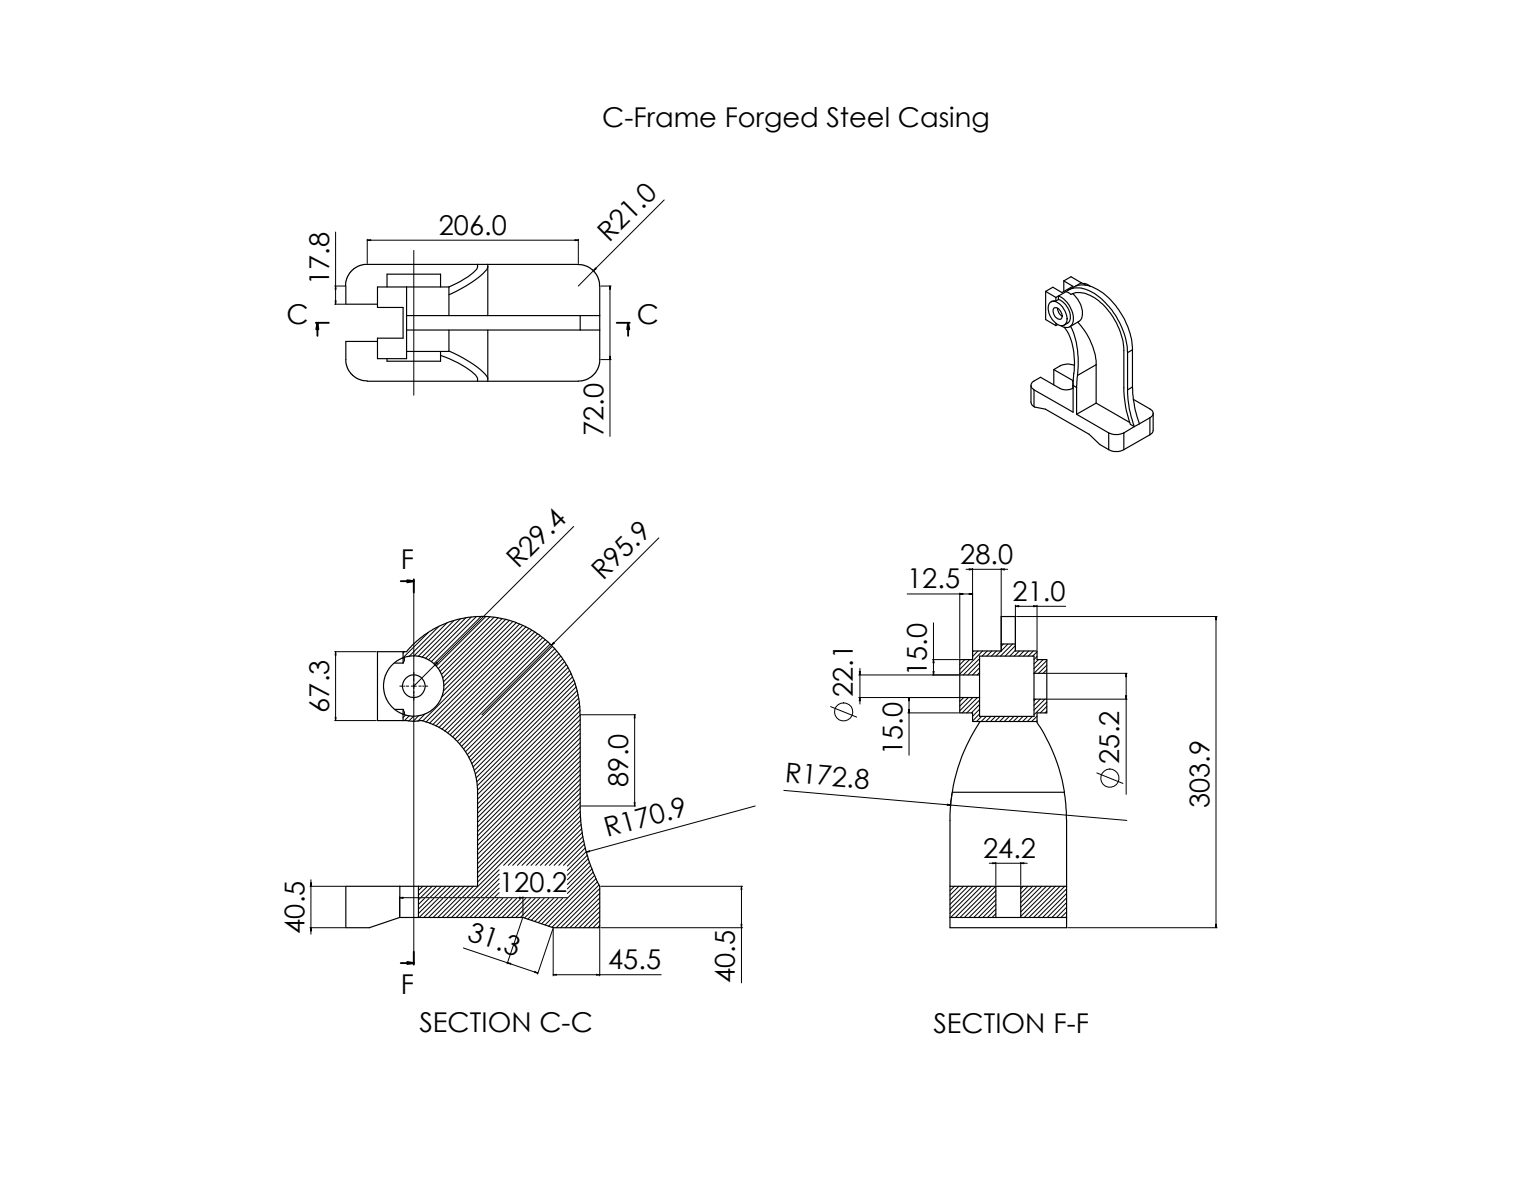
ISO-10303-21;
HEADER;
FILE_DESCRIPTION (('STEP AP214'),
    '1' );
FILE_NAME ('C-Frame Forged Steel Casing.step',
    '2026-10-21T18:33:49',
    ( '' ),
    ( '' ),
    'SwSTEP 2.0',
    'SolidWorks 2025',
    '' );
FILE_SCHEMA (( 'AUTOMOTIVE_DESIGN' ));
ENDSEC;

DATA;
#4=VERTEX_POINT ( 'NONE', #5573 ) ;
#12=DIRECTION ( 'NONE',  ( -0.000000000000000000, -0.000000000000000000, -1.000000000000000000 ) ) ;
#27=ADVANCED_FACE ( 'NONE', ( #4362 ), #9999, .F. ) ;
#28=VECTOR ( 'NONE', #11841, 1000.000000000000000 ) ;
#45=AXIS2_PLACEMENT_3D ( 'NONE', #14996, #2189, #7901 ) ;
#46=ORIENTED_EDGE ( 'NONE', *, *, #11434, .F. ) ;
#52=DIRECTION ( 'NONE',  ( -1.000000000000000000, -0.000000000000000000, -0.000000000000000000 ) ) ;
#63=CARTESIAN_POINT ( 'NONE',  ( -9.730036491473859073, 24.55694320255973651, 41.56001028271458608 ) ) ;
#65=ORIENTED_EDGE ( 'NONE', *, *, #13144, .F. ) ;
#81=ADVANCED_FACE ( 'NONE', ( #3143 ), #14460, .T. ) ;
#90=DIRECTION ( 'NONE',  ( -0.000000000000000000, 0.000000000000000000, -1.000000000000000000 ) ) ;
#91=LINE ( 'NONE', #5786, #7353 ) ;
#111=AXIS2_PLACEMENT_3D ( 'NONE', #807, #12215, #17823 ) ;
#116=EDGE_CURVE ( 'NONE', #6374, #8001, #17153, .T. ) ;
#139=CARTESIAN_POINT ( 'NONE',  ( -127.5926225674731711, 57.88796029049329661, -26.35917033480641436 ) ) ;
#144=ADVANCED_FACE ( 'NONE', ( #11916 ), #17609, .T. ) ;
#164=DIRECTION ( 'NONE',  ( -1.000000000000000000, 0.000000000000000000, 0.000000000000000000 ) ) ;
#170=FACE_OUTER_BOUND ( 'NONE', #6777, .T. ) ;
#173=VECTOR ( 'NONE', #14749, 1000.000000000000000 ) ;
#176=DIRECTION ( 'NONE',  ( 0.000000000000000000, 1.000000000000000000, 0.000000000000000000 ) ) ;
#177=ORIENTED_EDGE ( 'NONE', *, *, #14769, .T. ) ;
#183=CARTESIAN_POINT ( 'NONE',  ( -70.85175816390371040, -141.5628872026273086, -18.23991632971910803 ) ) ;
#186=CARTESIAN_POINT ( 'NONE',  ( 49.38736944425944841, -141.5628872026273086, -57.00000000000000000 ) ) ;
#188=DIRECTION ( 'NONE',  ( 0.000000000000000000, 0.000000000000000000, 1.000000000000000000 ) ) ;
#203=FACE_OUTER_BOUND ( 'NONE', #17910, .T. ) ;
#204=FACE_OUTER_BOUND ( 'NONE', #12195, .T. ) ;
#205=CARTESIAN_POINT ( 'NONE',  ( -64.09025127992788384, 50.58224449241410525, 35.00000000000000000 ) ) ;
#225=ORIENTED_EDGE ( 'NONE', *, *, #7011, .F. ) ;
#229=EDGE_CURVE ( 'NONE', #6748, #3936, #16550, .T. ) ;
#231=ORIENTED_EDGE ( 'NONE', *, *, #17262, .F. ) ;
#234=DIRECTION ( 'NONE',  ( 0.000000000000000000, 0.000000000000000000, 1.000000000000000000 ) ) ;
#236=ORIENTED_EDGE ( 'NONE', *, *, #5271, .F. ) ;
#241=ORIENTED_EDGE ( 'NONE', *, *, #15088, .F. ) ;
#244=EDGE_CURVE ( 'NONE', #4575, #11504, #16586, .T. ) ;
#255=EDGE_CURVE ( 'NONE', #17238, #6285, #13006, .T. ) ;
#263=ORIENTED_EDGE ( 'NONE', *, *, #18181, .T. ) ;
#266=CARTESIAN_POINT ( 'NONE',  ( -37.39678785461407529, 56.02900023377289074, 23.03959524935876857 ) ) ;
#268=DIRECTION ( 'NONE',  ( -0.000000000000000000, -0.000000000000000000, -1.000000000000000000 ) ) ;
#270=ORIENTED_EDGE ( 'NONE', *, *, #16707, .F. ) ;
#271=CARTESIAN_POINT ( 'NONE',  ( -66.92930002414082935, 60.44851893123529152, 25.00000000000000000 ) ) ;
#284=DIRECTION ( 'NONE',  ( 0.000000000000000000, 0.000000000000000000, 1.000000000000000000 ) ) ;
#293=VERTEX_POINT ( 'NONE', #8174 ) ;
#299=VERTEX_POINT ( 'NONE', #17149 ) ;
#301=DIRECTION ( 'NONE',  ( 0.000000000000000000, 0.000000000000000000, -1.000000000000000000 ) ) ;
#302=CARTESIAN_POINT ( 'NONE',  ( 105.4583593777967963, -32.62665103886256190, -7.000000000000010658 ) ) ;
#306=ORIENTED_EDGE ( 'NONE', *, *, #1227, .F. ) ;
#318=AXIS2_PLACEMENT_3D ( 'NONE', #739, #6431, #16426 ) ;
#325=CARTESIAN_POINT ( 'NONE',  ( -69.66239992860627694, 84.22855780814606419, 37.50000000000000000 ) ) ;
#330=ORIENTED_EDGE ( 'NONE', *, *, #16668, .T. ) ;
#331=EDGE_CURVE ( 'NONE', #1479, #11856, #14263, .T. ) ;
#337=AXIS2_PLACEMENT_3D ( 'NONE', #17527, #14630, #13242 ) ;
#355=FACE_OUTER_BOUND ( 'NONE', #8735, .T. ) ;
#357=CARTESIAN_POINT ( 'NONE',  ( -57.08002265617300708, 84.22855780814606419, 37.50000000000000000 ) ) ;
#367=CARTESIAN_POINT ( 'NONE',  ( -66.14751942900640813, 58.73266222548429027, 25.00000000000001066 ) ) ;
#375=CYLINDRICAL_SURFACE ( 'NONE', #9052, 85.91469608272775815 ) ;
#378=CARTESIAN_POINT ( 'NONE',  ( -71.20965894365861004, 109.9770744052236324, 22.40029077787859890 ) ) ;
#384=DIRECTION ( 'NONE',  ( -0.000000000000000000, 1.000000000000000000, -1.200240087506842815E-16 ) ) ;
#390=DIRECTION ( 'NONE',  ( 0.000000000000000000, 0.000000000000000000, 1.000000000000000000 ) ) ;
#394=CIRCLE ( 'NONE', #2180, 3.999999999999982681 ) ;
#395=AXIS2_PLACEMENT_3D ( 'NONE', #4110, #9813, #15514 ) ;
#397=CARTESIAN_POINT ( 'NONE',  ( -50.06979403241810900, 50.58224449241409104, -26.91246033477409583 ) ) ;
#399=ORIENTED_EDGE ( 'NONE', *, *, #757, .T. ) ;
#412=AXIS2_PLACEMENT_3D ( 'NONE', #18211, #5379, #6987 ) ;
#414=EDGE_CURVE ( 'NONE', #2953, #996, #7597, .T. ) ;
#416=EDGE_CURVE ( 'NONE', #17198, #9318, #10399, .T. ) ;
#420=VECTOR ( 'NONE', #9508, 1000.000000000000000 ) ;
#426=DIRECTION ( 'NONE',  ( -0.000000000000000000, -0.000000000000000000, -1.000000000000000000 ) ) ;
#429=ORIENTED_EDGE ( 'NONE', *, *, #6145, .F. ) ;
#430=VECTOR ( 'NONE', #5454, 1000.000000000000000 ) ;
#433=CARTESIAN_POINT ( 'NONE',  ( 15.23320273812466574, -111.0842361345572158, 57.00000000000000000 ) ) ;
#443=( LENGTH_UNIT ( ) NAMED_UNIT ( * ) SI_UNIT ( .MILLI., .METRE. ) );
#452=AXIS2_PLACEMENT_3D ( 'NONE', #2320, #3822, #12451 ) ;
#457=EDGE_CURVE ( 'NONE', #3111, #2581, #12721, .T. ) ;
#468=EDGE_CURVE ( 'NONE', #18251, #15291, #12961, .T. ) ;
#476=DIRECTION ( 'NONE',  ( 0.000000000000000000, 0.000000000000000000, -1.000000000000000000 ) ) ;
#481=CARTESIAN_POINT ( 'NONE',  ( 113.3630170098442989, -111.0842361345572158, -3.000000000000000000 ) ) ;
#482=ORIENTED_EDGE ( 'NONE', *, *, #4046, .F. ) ;
#485=EDGE_CURVE ( 'NONE', #2052, #18444, #13583, .T. ) ;
#486=ORIENTED_EDGE ( 'NONE', *, *, #1405, .F. ) ;
#487=ADVANCED_FACE ( 'NONE', ( #16560 ), #14878, .T. ) ;
#491=CARTESIAN_POINT ( 'NONE',  ( -38.40665361001209988, 55.34834135440265612, -23.54080219878014546 ) ) ;
#492=CARTESIAN_POINT ( 'NONE',  ( -102.4618227840623774, -151.5628872026273086, 57.00000000000000000 ) ) ;
#496=CARTESIAN_POINT ( 'NONE',  ( 276.3098885457529832, -32.62665103886256190, 7.000000000000010658 ) ) ;
#503=ORIENTED_EDGE ( 'NONE', *, *, #14484, .F. ) ;
#504=ORIENTED_EDGE ( 'NONE', *, *, #2706, .T. ) ;
#505=VERTEX_POINT ( 'NONE', #2158 ) ;
#510=DIRECTION ( 'NONE',  ( -0.000000000000000000, 0.000000000000000000, 1.000000000000000000 ) ) ;
#523=EDGE_LOOP ( 'NONE', ( #7059, #9577, #8331, #14594 ) ) ;
#530=CARTESIAN_POINT ( 'NONE',  ( -66.63376473465912397, -19.34983604512935429, 57.00000000000000000 ) ) ;
#532=CARTESIAN_POINT ( 'NONE',  ( -67.59262256747319952, 110.5691553257988460, -30.35917033480640370 ) ) ;
#535=VERTEX_POINT ( 'NONE', #769 ) ;
#537=DIRECTION ( 'NONE',  ( 0.000000000000000000, 1.000000000000000000, 0.000000000000000000 ) ) ;
#543=ORIENTED_EDGE ( 'NONE', *, *, #11265, .T. ) ;
#546=DIRECTION ( 'NONE',  ( 1.000000000000000000, 0.000000000000000000, 0.000000000000000000 ) ) ;
#550=CARTESIAN_POINT ( 'NONE',  ( 124.5381772159375942, -151.5628872026272802, 57.00000000000000000 ) ) ;
#552=CARTESIAN_POINT ( 'NONE',  ( -86.44887054343442401, 84.22855780814606419, -15.00000000000000711 ) ) ;
#556=CARTESIAN_POINT ( 'NONE',  ( -76.09645744896180020, 61.84763831329342310, -26.96898856272271772 ) ) ;
#559=ORIENTED_EDGE ( 'NONE', *, *, #11791, .T. ) ;
#561=ADVANCED_FACE ( 'NONE', ( #13672, #6655 ), #7775, .T. ) ;
#565=VERTEX_POINT ( 'NONE', #10486 ) ;
#570=ADVANCED_FACE ( 'NONE', ( #7868 ), #12377, .F. ) ;
#573=VERTEX_POINT ( 'NONE', #14965 ) ;
#588=CARTESIAN_POINT ( 'NONE',  ( -127.5926225674731711, 57.88796029049329661, -22.35917033480642502 ) ) ;
#591=ORIENTED_EDGE ( 'NONE', *, *, #12155, .F. ) ;
#608=CARTESIAN_POINT ( 'NONE',  ( -66.46434123065944277, 108.9297695310272331, 25.00000000000000000 ) ) ;
#609=ORIENTED_EDGE ( 'NONE', *, *, #8356, .T. ) ;
#611=CARTESIAN_POINT ( 'NONE',  ( -67.59262256747319952, 110.5691553257988460, 26.35917033480641436 ) ) ;
#615=AXIS2_PLACEMENT_3D ( 'NONE', #18506, #12902, #11404 ) ;
#632=CARTESIAN_POINT ( 'NONE',  ( 15.23320273812466041, -46.83756720124470263, -57.00000000000000000 ) ) ;
#637=DIRECTION ( 'NONE',  ( -1.000000000000000000, -0.000000000000000000, -0.000000000000000000 ) ) ;
#656=CARTESIAN_POINT ( 'NONE',  ( -75.85991620623855169, 61.64845565236244340, -24.98030658468874066 ) ) ;
#661=AXIS2_PLACEMENT_3D ( 'NONE', #357, #3872, #9580 ) ;
#670=DIRECTION ( 'NONE',  ( -0.000000000000000000, 1.000000000000000000, -0.000000000000000000 ) ) ;
#678=EDGE_CURVE ( 'NONE', #17304, #14302, #10606, .T. ) ;
#679=CYLINDRICAL_SURFACE ( 'NONE', #15266, 180.8515291679561585 ) ;
#680=DIRECTION ( 'NONE',  ( 1.000000000000000000, 2.062304371594500494E-16, -0.000000000000000000 ) ) ;
#685=ORIENTED_EDGE ( 'NONE', *, *, #12458, .T. ) ;
#687=EDGE_CURVE ( 'NONE', #18482, #6976, #11196, .T. ) ;
#707=ORIENTED_EDGE ( 'NONE', *, *, #4942, .F. ) ;
#712=ADVANCED_FACE ( 'NONE', ( #1423 ), #18070, .F. ) ;
#713=CARTESIAN_POINT ( 'NONE',  ( 49.38736944425944841, -141.5628872026273086, -57.00000000000000000 ) ) ;
#721=ORIENTED_EDGE ( 'NONE', *, *, #229, .F. ) ;
#726=CARTESIAN_POINT ( 'NONE',  ( 5.233202738124663966, -15.18076580469977621, 54.12731639097741976 ) ) ;
#727=EDGE_CURVE ( 'NONE', #299, #9555, #15255, .T. ) ;
#739=CARTESIAN_POINT ( 'NONE',  ( -127.5926225674731711, 57.88796029049329661, 26.35917033480641436 ) ) ;
#741=PLANE ( 'NONE',  #2390 ) ;
#748=VERTEX_POINT ( 'NONE', #8151 ) ;
#752=CARTESIAN_POINT ( 'NONE',  ( -66.09157170483439359, 57.23989889526016839, 25.00000000000000711 ) ) ;
#757=EDGE_CURVE ( 'NONE', #8476, #13829, #13867, .T. ) ;
#758=CARTESIAN_POINT ( 'NONE',  ( -73.90024509548729270, 60.14960425286541579, -23.04802554496307820 ) ) ;
#769=CARTESIAN_POINT ( 'NONE',  ( -92.59262256747321373, 117.8748711238780373, -35.00000000000000000 ) ) ;
#777=LINE ( 'NONE', #16857, #3625 ) ;
#788=DIRECTION ( 'NONE',  ( 0.000000000000000000, 0.000000000000000000, 1.000000000000000000 ) ) ;
#791=CARTESIAN_POINT ( 'NONE',  ( -92.59262256747319952, 57.88796029049329661, -26.35917033480641436 ) ) ;
#798=DIRECTION ( 'NONE',  ( -0.000000000000000000, -0.000000000000000000, -1.000000000000000000 ) ) ;
#802=ADVANCED_FACE ( 'NONE', ( #10295 ), #10201, .F. ) ;
#804=CARTESIAN_POINT ( 'NONE',  ( -102.4618227840623774, -151.5628872026273086, -36.00000000000000000 ) ) ;
#806=ORIENTED_EDGE ( 'NONE', *, *, #924, .F. ) ;
#807=CARTESIAN_POINT ( 'NONE',  ( -57.08002265617300708, 84.22855780814606419, -35.00000000000000711 ) ) ;
#838=CARTESIAN_POINT ( 'NONE',  ( -64.09025127992788384, 50.58224449241410525, 35.00000000000000000 ) ) ;
#843=CARTESIAN_POINT ( 'NONE',  ( -123.4618227840623632, -151.5628872026273086, -18.23991632971910093 ) ) ;
#847=FACE_OUTER_BOUND ( 'NONE', #13419, .T. ) ;
#862=ORIENTED_EDGE ( 'NONE', *, *, #18382, .T. ) ;
#870=AXIS2_PLACEMENT_3D ( 'NONE', #11609, #12763, #7219 ) ;
#880=CARTESIAN_POINT ( 'NONE',  ( -123.4618227840623632, -111.0842361345572158, 57.00000000000000000 ) ) ;
#882=AXIS2_PLACEMENT_3D ( 'NONE', #13146, #12986, #164 ) ;
#883=CARTESIAN_POINT ( 'NONE',  ( -72.81448312412459245, 109.0309132574646469, -22.65846447477133196 ) ) ;
#885=VERTEX_POINT ( 'NONE', #5803 ) ;
#890=EDGE_CURVE ( 'NONE', #6749, #1925, #15737, .T. ) ;
#892=AXIS2_PLACEMENT_3D ( 'NONE', #1155, #10880, #1247 ) ;
#898=VECTOR ( 'NONE', #16815, 1000.000000000000000 ) ;
#902=B_SPLINE_CURVE_WITH_KNOTS ( 'NONE', 3,
 ( #11513, #2811, #7287, #2981 ),
 .UNSPECIFIED., .F., .F.,
 ( 4, 4 ),
 ( 0.000000000000000000, 0.002699315152504066541 ),
 .UNSPECIFIED. ) ;
#906=CARTESIAN_POINT ( 'NONE',  ( -67.59262256747319952, 110.5691553257988460, 30.35917033480640370 ) ) ;
#908=CARTESIAN_POINT ( 'NONE',  ( 9.543663295069050534, 56.41207303426870112, 7.000000000000010658 ) ) ;
#916=DIRECTION ( 'NONE',  ( -1.000000000000000000, 0.000000000000000000, -0.000000000000000000 ) ) ;
#924=EDGE_CURVE ( 'NONE', #6138, #3111, #9170, .T. ) ;
#927=CARTESIAN_POINT ( 'NONE',  ( -66.75350761719796822, 56.49772428296282811, 24.14382665953563745 ) ) ;
#929=CARTESIAN_POINT ( 'NONE',  ( -66.56081925660646448, 59.51305259755623212, -27.99999999999999645 ) ) ;
#931=EDGE_CURVE ( 'NONE', #505, #8038, #6442, .T. ) ;
#934=EDGE_CURVE ( 'NONE', #15744, #1208, #5522, .T. ) ;
#938=ORIENTED_EDGE ( 'NONE', *, *, #890, .F. ) ;
#946=DIRECTION ( 'NONE',  ( -0.000000000000000000, 0.000000000000000000, 1.000000000000000000 ) ) ;
#951=ADVANCED_FACE ( 'NONE', ( #5030 ), #13463, .F. ) ;
#963=CARTESIAN_POINT ( 'NONE',  ( -123.4618227840623632, -151.5628872026273086, 57.00000000000000000 ) ) ;
#982=VECTOR ( 'NONE', #13264, 1000.000000000000000 ) ;
#986=ORIENTED_EDGE ( 'NONE', *, *, #12489, .F. ) ;
#987=CARTESIAN_POINT ( 'NONE',  ( -74.24593559006332555, 108.0616442416786640, -23.22608149512904063 ) ) ;
#994=DIRECTION ( 'NONE',  ( -0.000000000000000000, -1.000000000000000000, -0.000000000000000000 ) ) ;
#996=VERTEX_POINT ( 'NONE', #13656 ) ;
#1007=CARTESIAN_POINT ( 'NONE',  ( -123.4618227840623632, -111.0842361345572158, 57.00000000000000000 ) ) ;
#1008=ORIENTED_EDGE ( 'NONE', *, *, #10694, .T. ) ;
#1010=CARTESIAN_POINT ( 'NONE',  ( -112.5926225674731995, 50.58224449241410525, 35.00000000000000000 ) ) ;
#1018=AXIS2_PLACEMENT_3D ( 'NONE', #18076, #8156, #2447 ) ;
#1021=FACE_OUTER_BOUND ( 'NONE', #2125, .T. ) ;
#1023=VECTOR ( 'NONE', #12613, 1000.000000000000000 ) ;
#1026=CARTESIAN_POINT ( 'NONE',  ( 103.5381772159376084, -151.5628872026272802, 57.00000000000000000 ) ) ;
#1027=AXIS2_PLACEMENT_3D ( 'NONE', #13141, #17251, #1911 ) ;
#1029=CARTESIAN_POINT ( 'NONE',  ( -67.37336793441032512, 56.72162401922281560, 22.91103267187422787 ) ) ;
#1038=CARTESIAN_POINT ( 'NONE',  ( -0.000000000000000000, -111.0842361345572158, -3.000000000000000000 ) ) ;
#1040=ORIENTED_EDGE ( 'NONE', *, *, #11176, .F. ) ;
#1041=EDGE_CURVE ( 'NONE', #13411, #11585, #10588, .T. ) ;
#1049=ORIENTED_EDGE ( 'NONE', *, *, #15194, .T. ) ;
#1054=AXIS2_PLACEMENT_3D ( 'NONE', #5183, #18105, #10990 ) ;
#1059=CARTESIAN_POINT ( 'NONE',  ( -64.09025127992789805, 117.8748711238780089, 7.000000000000010658 ) ) ;
#1063=EDGE_CURVE ( 'NONE', #3060, #4, #4507, .T. ) ;
#1067=VECTOR ( 'NONE', #16551, 1000.000000000000000 ) ;
#1069=CARTESIAN_POINT ( 'NONE',  ( -112.5926225674731853, 50.58224449241410525, 15.00000000000004796 ) ) ;
#1072=DIRECTION ( 'NONE',  ( 0.000000000000000000, 0.000000000000000000, 1.000000000000000000 ) ) ;
#1080=EDGE_LOOP ( 'NONE', ( #7717, #7540 ) ) ;
#1083=VECTOR ( 'NONE', #15801, 1000.000000000000000 ) ;
#1084=VECTOR ( 'NONE', #5911, 1000.000000000000000 ) ;
#1086=CARTESIAN_POINT ( 'NONE',  ( 9.543663295069050534, 56.41207303426870112, -7.000000000000010658 ) ) ;
#1091=ORIENTED_EDGE ( 'NONE', *, *, #16945, .T. ) ;
#1092=CARTESIAN_POINT ( 'NONE',  ( -100.4870060002411805, -151.5628872026273086, 18.23991632971911514 ) ) ;
#1096=CARTESIAN_POINT ( 'NONE',  ( -75.82627924895463423, 106.8366279053472283, -27.81200583293166417 ) ) ;
#1104=ORIENTED_EDGE ( 'NONE', *, *, #9720, .F. ) ;
#1105=DIRECTION ( 'NONE',  ( -0.9475106458593564041, 0.3197242186372270534, -0.000000000000000000 ) ) ;
#1113=CARTESIAN_POINT ( 'NONE',  ( 5.233202738124664855, -19.34983604512936495, -54.79921157549230770 ) ) ;
#1114=CARTESIAN_POINT ( 'NONE',  ( -6.009442422294567265, 35.67642109510119752, 36.02332778080708664 ) ) ;
#1123=PLANE ( 'NONE',  #1879 ) ;
#1124=LINE ( 'NONE', #7948, #12683 ) ;
#1127=CARTESIAN_POINT ( 'NONE',  ( -45.07766827056850190, 51.92519128693054142, 25.99195503995988688 ) ) ;
#1132=CARTESIAN_POINT ( 'NONE',  ( -123.4618227840623632, -151.5628872026273086, 57.00000000000000000 ) ) ;
#1133=EDGE_LOOP ( 'NONE', ( #5557, #3035, #10608, #2937 ) ) ;
#1135=DIRECTION ( 'NONE',  ( -1.000000000000000000, 0.000000000000000000, 0.000000000000000000 ) ) ;
#1141=DIRECTION ( 'NONE',  ( 0.000000000000000000, 0.000000000000000000, 1.000000000000000000 ) ) ;
#1151=PLANE ( 'NONE',  #16206 ) ;
#1153=EDGE_CURVE ( 'NONE', #16485, #3472, #5228, .T. ) ;
#1155=CARTESIAN_POINT ( 'NONE',  ( -102.4618227840623774, -111.0842361345572158, 36.00000000000000711 ) ) ;
#1163=EDGE_CURVE ( 'NONE', #13829, #10929, #1213, .T. ) ;
#1170=CARTESIAN_POINT ( 'NONE',  ( -5.374518711846989483, 34.99587063685016375, -36.39809049692809850 ) ) ;
#1172=ORIENTED_EDGE ( 'NONE', *, *, #11434, .T. ) ;
#1173=EDGE_CURVE ( 'NONE', #9439, #10991, #7622, .T. ) ;
#1175=CARTESIAN_POINT ( 'NONE',  ( -67.59262256747319952, 111.6514400295689171, 22.50837044127971254 ) ) ;
#1190=EDGE_LOOP ( 'NONE', ( #11318, #6672, #1682, #10970 ) ) ;
#1200=CARTESIAN_POINT ( 'NONE',  ( -75.73736374306625407, 106.9102428511424279, 24.71466311077380951 ) ) ;
#1205=DIRECTION ( 'NONE',  ( -2.062304371594500494E-16, 1.000000000000000000, 2.385018538676381657E-32 ) ) ;
#1208=VERTEX_POINT ( 'NONE', #5869 ) ;
#1210=ORIENTED_EDGE ( 'NONE', *, *, #3545, .T. ) ;
#1213=LINE ( 'NONE', #16630, #7917 ) ;
#1216=ORIENTED_EDGE ( 'NONE', *, *, #17723, .T. ) ;
#1218=CARTESIAN_POINT ( 'NONE',  ( -57.08002265617300708, 84.22855780814606419, 25.00000000000000355 ) ) ;
#1227=EDGE_CURVE ( 'NONE', #17762, #13685, #17235, .T. ) ;
#1232=VECTOR ( 'NONE', #3529, 1000.000000000000000 ) ;
#1240=CARTESIAN_POINT ( 'NONE',  ( -31.03642545851250745, 84.22855780814606419, -47.49999999999999289 ) ) ;
#1245=CIRCLE ( 'NONE', #5995, 11.04359719766049430 ) ;
#1247=DIRECTION ( 'NONE',  ( 6.608470384673552010E-16, 0.000000000000000000, -1.000000000000000000 ) ) ;
#1253=VERTEX_POINT ( 'NONE', #10094 ) ;
#1255=CIRCLE ( 'NONE', #12295, 95.91469608272775815 ) ;
#1258=DIRECTION ( 'NONE',  ( 0.000000000000000000, 8.876422075684827903E-15, -1.000000000000000000 ) ) ;
#1259=ORIENTED_EDGE ( 'NONE', *, *, #8733, .F. ) ;
#1263=CARTESIAN_POINT ( 'NONE',  ( -0.3548237229735157761, 28.74729804758344542, -39.59865668900319946 ) ) ;
#1267=CARTESIAN_POINT ( 'NONE',  ( 276.3098885457529832, -32.62665103886256190, -3.000000000000000000 ) ) ;
#1272=CARTESIAN_POINT ( 'NONE',  ( -75.66320186394305836, 106.9708331287094580, -24.59982859766222418 ) ) ;
#1278=DIRECTION ( 'NONE',  ( -0.9475106458593564041, -0.3197242186372270534, -0.000000000000000000 ) ) ;
#1286=ORIENTED_EDGE ( 'NONE', *, *, #7547, .T. ) ;
#1288=CIRCLE ( 'NONE', #16496, 172.7605492041889192 ) ;
#1293=CARTESIAN_POINT ( 'NONE',  ( 113.3630170098442989, -111.0842361345572158, -7.000000000000010658 ) ) ;
#1300=CARTESIAN_POINT ( 'NONE',  ( -50.06979403241810900, 50.58224449241409104, -26.91246033477409583 ) ) ;
#1302=CARTESIAN_POINT ( 'NONE',  ( 14.89878123376213814, -10.86838903421133296, 53.26686714696702296 ) ) ;
#1316=CARTESIAN_POINT ( 'NONE',  ( -67.59262256747315689, 117.8748711238780373, 15.00000000000006040 ) ) ;
#1347=EDGE_LOOP ( 'NONE', ( #13122, #1894, #1210, #14682 ) ) ;
#1356=ORIENTED_EDGE ( 'NONE', *, *, #11337, .F. ) ;
#1360=CARTESIAN_POINT ( 'NONE',  ( 5.233202738124664855, -46.83756720124469553, -57.00000000000000000 ) ) ;
#1363=ORIENTED_EDGE ( 'NONE', *, *, #8009, .T. ) ;
#1367=DIRECTION ( 'NONE',  ( 1.000000000000000000, 0.000000000000000000, 0.000000000000000000 ) ) ;
#1368=ORIENTED_EDGE ( 'NONE', *, *, #7763, .T. ) ;
#1370=FACE_OUTER_BOUND ( 'NONE', #10235, .T. ) ;
#1377=LINE ( 'NONE', #12792, #2573 ) ;
#1379=ORIENTED_EDGE ( 'NONE', *, *, #12840, .T. ) ;
#1382=CARTESIAN_POINT ( 'NONE',  ( -57.08002265617300708, 84.22855780814606419, 25.00000000000000355 ) ) ;
#1383=DIRECTION ( 'NONE',  ( -0.000000000000000000, -0.000000000000000000, -1.000000000000000000 ) ) ;
#1390=CARTESIAN_POINT ( 'NONE',  ( -32.10604320681301971, 43.68747662467802684, -31.38471465307124220 ) ) ;
#1391=CARTESIAN_POINT ( 'NONE',  ( 15.23320273812465864, -15.06249217057395917, 54.10825519012411178 ) ) ;
#1392=ORIENTED_EDGE ( 'NONE', *, *, #1153, .T. ) ;
#1405=EDGE_CURVE ( 'NONE', #14435, #10632, #13014, .T. ) ;
#1407=EDGE_CURVE ( 'NONE', #8420, #15506, #15340, .T. ) ;
#1410=CARTESIAN_POINT ( 'NONE',  ( -67.59262256747319952, 106.9211863004615140, -28.00000000000000355 ) ) ;
#1423=FACE_OUTER_BOUND ( 'NONE', #1747, .T. ) ;
#1430=LINE ( 'NONE', #4140, #6605 ) ;
#1445=CARTESIAN_POINT ( 'NONE',  ( -1.560979369245516946, 30.36679981511084137, -38.79937448922311205 ) ) ;
#1447=ORIENTED_EDGE ( 'NONE', *, *, #1173, .T. ) ;
#1456=EDGE_CURVE ( 'NONE', #996, #10176, #9633, .T. ) ;
#1458=ORIENTED_EDGE ( 'NONE', *, *, #17275, .F. ) ;
#1459=AXIS2_PLACEMENT_3D ( 'NONE', #9644, #6931, #1135 ) ;
#1462=VERTEX_POINT ( 'NONE', #11325 ) ;
#1471=CARTESIAN_POINT ( 'NONE',  ( 8.585741852500916593, 13.02923129865365048, 46.30804433544984988 ) ) ;
#1474=DIRECTION ( 'NONE',  ( -0.000000000000000000, -0.000000000000000000, -1.000000000000000000 ) ) ;
#1479=VERTEX_POINT ( 'NONE', #13094 ) ;
#1489=DIRECTION ( 'NONE',  ( -1.000000000000000000, 0.000000000000000000, 0.000000000000000000 ) ) ;
#1502=CARTESIAN_POINT ( 'NONE',  ( 15.23320273812466041, -46.83756720124470263, 57.00000000000000000 ) ) ;
#1507=EDGE_CURVE ( 'NONE', #573, #17254, #15800, .T. ) ;
#1521=DIRECTION ( 'NONE',  ( -1.558623840612994987E-16, -1.000000000000000000, 0.000000000000000000 ) ) ;
#1530=CIRCLE ( 'NONE', #16093, 20.99999999999998934 ) ;
#1531=ORIENTED_EDGE ( 'NONE', *, *, #11525, .T. ) ;
#1546=AXIS2_PLACEMENT_3D ( 'NONE', #7135, #17137, #4325 ) ;
#1554=DIRECTION ( 'NONE',  ( -0.000000000000000000, -0.000000000000000000, 1.000000000000000000 ) ) ;
#1556=EDGE_LOOP ( 'NONE', ( #15169, #11479, #6546, #10377 ) ) ;
#1588=VECTOR ( 'NONE', #2520, 1000.000000000000000 ) ;
#1596=ORIENTED_EDGE ( 'NONE', *, *, #8148, .T. ) ;
#1599=EDGE_CURVE ( 'NONE', #11975, #10530, #91, .T. ) ;
#1602=CARTESIAN_POINT ( 'NONE',  ( 103.5381772159376084, 0.000000000000000000, 36.00000000000000711 ) ) ;
#1606=ORIENTED_EDGE ( 'NONE', *, *, #11097, .F. ) ;
#1608=ORIENTED_EDGE ( 'NONE', *, *, #9877, .T. ) ;
#1611=ORIENTED_EDGE ( 'NONE', *, *, #16336, .F. ) ;
#1618=AXIS2_PLACEMENT_3D ( 'NONE', #1086, #2575, #8275 ) ;
#1628=ADVANCED_FACE ( 'NONE', ( #6320 ), #16244, .F. ) ;
#1634=DIRECTION ( 'NONE',  ( -1.982541115402065702E-15, 0.000000000000000000, -1.000000000000000000 ) ) ;
#1639=EDGE_LOOP ( 'NONE', ( #3526, #4049 ) ) ;
#1640=EDGE_CURVE ( 'NONE', #3309, #2052, #3169, .T. ) ;
#1646=DIRECTION ( 'NONE',  ( -1.000000000000000000, 0.000000000000000000, 0.000000000000000000 ) ) ;
#1682=ORIENTED_EDGE ( 'NONE', *, *, #17517, .T. ) ;
#1691=LINE ( 'NONE', #14251, #2758 ) ;
#1693=FACE_OUTER_BOUND ( 'NONE', #14514, .T. ) ;
#1700=ADVANCED_FACE ( 'NONE', ( #8966 ), #3247, .F. ) ;
#1705=EDGE_CURVE ( 'NONE', #9559, #15506, #7461, .T. ) ;
#1708=VERTEX_POINT ( 'NONE', #13355 ) ;
#1710=ADVANCED_FACE ( 'NONE', ( #355 ), #6044, .F. ) ;
#1724=LINE ( 'NONE', #7429, #16218 ) ;
#1744=EDGE_LOOP ( 'NONE', ( #2481, #4950, #13639, #5885 ) ) ;
#1747=EDGE_LOOP ( 'NONE', ( #12529, #685, #8352, #12835 ) ) ;
#1749=CARTESIAN_POINT ( 'NONE',  ( -66.21742401348355145, 112.1398742197459910, -27.07089588484168985 ) ) ;
#1750=LINE ( 'NONE', #17362, #12354 ) ;
#1753=EDGE_LOOP ( 'NONE', ( #14207, #862, #15105, #13118, #7710, #9924 ) ) ;
#1755=CARTESIAN_POINT ( 'NONE',  ( -64.09025127992788384, 50.58224449241410525, 35.00000000000000000 ) ) ;
#1762=EDGE_CURVE ( 'NONE', #12741, #9327, #15124, .T. ) ;
#1771=LINE ( 'NONE', #7479, #8037 ) ;
#1773=DIRECTION ( 'NONE',  ( -0.000000000000000000, -0.000000000000000000, -1.000000000000000000 ) ) ;
#1785=CARTESIAN_POINT ( 'NONE',  ( -46.03642545851251100, 84.22855780814606419, 37.50000000000000000 ) ) ;
#1787=VECTOR ( 'NONE', #3639, 1000.000000000000000 ) ;
#1792=CARTESIAN_POINT ( 'NONE',  ( 95.45835937779683888, -32.62665103886256190, 7.000000000000010658 ) ) ;
#1814=DIRECTION ( 'NONE',  ( -1.000000000000000000, 0.000000000000000000, 0.000000000000000000 ) ) ;
#1816=VECTOR ( 'NONE', #7709, 1000.000000000000000 ) ;
#1817=VECTOR ( 'NONE', #1554, 1000.000000000000000 ) ;
#1824=LINE ( 'NONE', #11748, #28 ) ;
#1841=ADVANCED_FACE ( 'NONE', ( #4611 ), #16906, .F. ) ;
#1842=AXIS2_PLACEMENT_3D ( 'NONE', #6115, #798, #17622 ) ;
#1849=AXIS2_PLACEMENT_3D ( 'NONE', #2031, #2124, #12150 ) ;
#1850=AXIS2_PLACEMENT_3D ( 'NONE', #5958, #8695, #14315 ) ;
#1852=EDGE_CURVE ( 'NONE', #7351, #2768, #9801, .T. ) ;
#1858=ORIENTED_EDGE ( 'NONE', *, *, #457, .T. ) ;
#1877=PLANE ( 'NONE',  #17077 ) ;
#1879=AXIS2_PLACEMENT_3D ( 'NONE', #18343, #2618, #8418 ) ;
#1884=DIRECTION ( 'NONE',  ( -1.000000000000000000, -0.000000000000000000, -0.000000000000000000 ) ) ;
#1885=ORIENTED_EDGE ( 'NONE', *, *, #8517, .T. ) ;
#1888=CONICAL_SURFACE ( 'NONE', #7865, 3.999999999999982681, 1.029744258676651203 ) ;
#1893=LINE ( 'NONE', #9372, #7837 ) ;
#1894=ORIENTED_EDGE ( 'NONE', *, *, #10650, .T. ) ;
#1895=VERTEX_POINT ( 'NONE', #5999 ) ;
#1896=B_SPLINE_CURVE_WITH_KNOTS ( 'NONE', 3,
 ( #17852, #5031, #10745, #16439, #13657, #16538, #3740, #2321, #13743, #11137, #6820, #12539, #15232, #18237, #8522, #9732, #7107, #17010 ),
 .UNSPECIFIED., .F., .F.,
 ( 4, 2, 2, 2, 2, 2, 2, 2, 4 ),
 ( 0.002699315152504171492, 0.004615533240672466987, 0.005573642284756619505, 0.006531751328840772891, 0.007489860372924925409, 0.008447969417009077928, 0.008927023939051153753, 0.009406078461093231313, 0.01036418750517741419 ),
 .UNSPECIFIED. ) ;
#1897=LINE ( 'NONE', #7605, #14378 ) ;
#1900=CYLINDRICAL_SURFACE ( 'NONE', #17107, 29.36884788726140627 ) ;
#1904=FACE_OUTER_BOUND ( 'NONE', #6363, .T. ) ;
#1905=CIRCLE ( 'NONE', #16530, 85.91469608272775815 ) ;
#1907=CIRCLE ( 'NONE', #111, 26.04359719766049608 ) ;
#1911=DIRECTION ( 'NONE',  ( 1.000000000000000000, 0.000000000000000000, 0.000000000000000000 ) ) ;
#1914=CIRCLE ( 'NONE', #15049, 12.58237727243326987 ) ;
#1916=AXIS2_PLACEMENT_3D ( 'NONE', #9758, #16562, #12379 ) ;
#1922=VERTEX_POINT ( 'NONE', #3129 ) ;
#1925=VERTEX_POINT ( 'NONE', #1300 ) ;
#1927=CARTESIAN_POINT ( 'NONE',  ( -92.59262256747321373, 117.8748711238780373, 35.00000000000000000 ) ) ;
#1932=AXIS2_PLACEMENT_3D ( 'NONE', #13369, #17851, #546 ) ;
#1939=LINE ( 'NONE', #7646, #420 ) ;
#1947=CARTESIAN_POINT ( 'NONE',  ( -70.85175816390371040, -141.5628872026273086, 18.23991632971911514 ) ) ;
#1951=VERTEX_POINT ( 'NONE', #15841 ) ;
#1957=ORIENTED_EDGE ( 'NONE', *, *, #14986, .T. ) ;
#1959=ORIENTED_EDGE ( 'NONE', *, *, #1153, .F. ) ;
#1962=AXIS2_PLACEMENT_3D ( 'NONE', #4693, #3032, #13131 ) ;
#1966=DIRECTION ( 'NONE',  ( -1.000000000000000000, 0.000000000000000000, 0.000000000000000000 ) ) ;
#1969=EDGE_CURVE ( 'NONE', #3472, #8476, #8196, .T. ) ;
#1974=CARTESIAN_POINT ( 'NONE',  ( -36.57592446955339227, 45.96055548693809101, -29.96385110796869000 ) ) ;
#1975=CARTESIAN_POINT ( 'NONE',  ( -75.82624405736112294, 61.62045879897588918, -27.81207011136935847 ) ) ;
#1987=ORIENTED_EDGE ( 'NONE', *, *, #12238, .T. ) ;
#2008=DIRECTION ( 'NONE',  ( -1.000000000000000000, 0.000000000000000000, 0.000000000000000000 ) ) ;
#2024=LINE ( 'NONE', #10364, #11191 ) ;
#2029=CARTESIAN_POINT ( 'NONE',  ( 276.3098885457529832, -32.62665103886256190, 7.000000000000010658 ) ) ;
#2031=CARTESIAN_POINT ( 'NONE',  ( -57.08002265617300708, 84.22855780814606419, 2.999999999999999112 ) ) ;
#2034=DIRECTION ( 'NONE',  ( 0.000000000000000000, 0.000000000000000000, 1.000000000000000000 ) ) ;
#2035=DIRECTION ( 'NONE',  ( 0.000000000000000000, 0.000000000000000000, 1.000000000000000000 ) ) ;
#2036=ORIENTED_EDGE ( 'NONE', *, *, #10317, .F. ) ;
#2042=DIRECTION ( 'NONE',  ( 1.000000000000000000, 0.000000000000000000, 0.000000000000000000 ) ) ;
#2047=DIRECTION ( 'NONE',  ( 1.000000000000000000, 0.000000000000000000, 0.000000000000000000 ) ) ;
#2052=VERTEX_POINT ( 'NONE', #3668 ) ;
#2056=CARTESIAN_POINT ( 'NONE',  ( -76.14069299065937457, 61.88532069570636907, -26.17446772214336548 ) ) ;
#2058=VECTOR ( 'NONE', #2684, 1000.000000000000000 ) ;
#2062=EDGE_LOOP ( 'NONE', ( #14474, #14620, #14701, #12280, #10684 ) ) ;
#2063=ADVANCED_FACE ( 'NONE', ( #6369 ), #7694, .F. ) ;
#2065=ADVANCED_FACE ( 'NONE', ( #3852 ), #1151, .F. ) ;
#2068=CARTESIAN_POINT ( 'NONE',  ( -57.08002265617300708, 84.22855780814606419, 37.50000000000000000 ) ) ;
#2080=CARTESIAN_POINT ( 'NONE',  ( -66.30216873316086890, 111.8377431448113555, 25.00000000000000355 ) ) ;
#2085=ADVANCED_FACE ( 'NONE', ( #6335 ), #12064, .T. ) ;
#2099=ORIENTED_EDGE ( 'NONE', *, *, #4636, .F. ) ;
#2102=VERTEX_POINT ( 'NONE', #13558 ) ;
#2106=DIRECTION ( 'NONE',  ( 0.000000000000000000, 0.000000000000000000, 1.000000000000000000 ) ) ;
#2110=CIRCLE ( 'NONE', #615, 85.91469608272775815 ) ;
#2111=VECTOR ( 'NONE', #3517, 1000.000000000000000 ) ;
#2120=AXIS2_PLACEMENT_3D ( 'NONE', #3968, #8182, #13901 ) ;
#2124=DIRECTION ( 'NONE',  ( 0.000000000000000000, -0.000000000000000000, -1.000000000000000000 ) ) ;
#2125=EDGE_LOOP ( 'NONE', ( #1987, #12915, #5110, #5381 ) ) ;
#2129=CYLINDRICAL_SURFACE ( 'NONE', #318, 3.999999999999989786 ) ;
#2139=CARTESIAN_POINT ( 'NONE',  ( 276.3098885457529832, -32.62665103886256190, 3.000000000000000000 ) ) ;
#2146=CARTESIAN_POINT ( 'NONE',  ( -74.71885885752763556, 60.74579698922836712, -23.55577225783097362 ) ) ;
#2148=VERTEX_POINT ( 'NONE', #1026 ) ;
#2158=CARTESIAN_POINT ( 'NONE',  ( -102.4618227840623774, -111.0842361345572158, 57.00000000000000000 ) ) ;
#2162=ORIENTED_EDGE ( 'NONE', *, *, #7545, .T. ) ;
#2164=FACE_OUTER_BOUND ( 'NONE', #1556, .T. ) ;
#2172=ORIENTED_EDGE ( 'NONE', *, *, #7203, .F. ) ;
#2176=DIRECTION ( 'NONE',  ( -1.000000000000000000, -0.000000000000000000, -0.000000000000000000 ) ) ;
#2177=VERTEX_POINT ( 'NONE', #12160 ) ;
#2180=AXIS2_PLACEMENT_3D ( 'NONE', #6764, #8165, #1072 ) ;
#2182=EDGE_CURVE ( 'NONE', #10531, #9679, #13248, .T. ) ;
#2187=DIRECTION ( 'NONE',  ( 0.000000000000000000, 0.000000000000000000, 1.000000000000000000 ) ) ;
#2188=ORIENTED_EDGE ( 'NONE', *, *, #9489, .F. ) ;
#2189=DIRECTION ( 'NONE',  ( -1.000000000000000000, -0.000000000000000000, -0.000000000000000000 ) ) ;
#2193=LINE ( 'NONE', #5080, #16443 ) ;
#2199=CARTESIAN_POINT ( 'NONE',  ( -66.09703808151903104, 109.8904997453310557, 24.99999999999999645 ) ) ;
#2207=LINE ( 'NONE', #7920, #1023 ) ;
#2212=CARTESIAN_POINT ( 'NONE',  ( 3.839371739003430761, -5.119679209322452351, 51.89990490011624047 ) ) ;
#2213=FACE_OUTER_BOUND ( 'NONE', #9873, .T. ) ;
#2219=CARTESIAN_POINT ( 'NONE',  ( -67.59262256747317110, 57.88796029049329661, 26.35917033480641436 ) ) ;
#2225=CARTESIAN_POINT ( 'NONE',  ( -57.08002265617300708, 84.22855780814606419, -28.00000000000000355 ) ) ;
#2232=VECTOR ( 'NONE', #13767, 1000.000000000000000 ) ;
#2240=CARTESIAN_POINT ( 'NONE',  ( -66.17391212418095847, 57.96819926477352425, -28.00000000000000000 ) ) ;
#2256=DIRECTION ( 'NONE',  ( -1.000000000000000000, -0.000000000000000000, -0.000000000000000000 ) ) ;
#2267=ORIENTED_EDGE ( 'NONE', *, *, #3675, .F. ) ;
#2272=VERTEX_POINT ( 'NONE', #1316 ) ;
#2273=ADVANCED_FACE ( 'NONE', ( #5594 ), #8518, .T. ) ;
#2284=CARTESIAN_POINT ( 'NONE',  ( -71.65892208273831443, 109.7273330359258665, -22.44256693161642247 ) ) ;
#2292=ADVANCED_FACE ( 'NONE', ( #10008 ), #15431, .F. ) ;
#2300=CARTESIAN_POINT ( 'NONE',  ( 9.543663295069050534, 56.41207303426870112, 7.000000000000010658 ) ) ;
#2302=ORIENTED_EDGE ( 'NONE', *, *, #14625, .T. ) ;
#2303=CARTESIAN_POINT ( 'NONE',  ( 105.4583593777968105, 56.41207303426870112, 7.000000000000010658 ) ) ;
#2306=CARTESIAN_POINT ( 'NONE',  ( -23.67723694629486531, 50.34933454821165810, 27.07273111978159008 ) ) ;
#2308=ADVANCED_FACE ( 'NONE', ( #5510, #11234 ), #16920, .F. ) ;
#2316=ORIENTED_EDGE ( 'NONE', *, *, #17517, .F. ) ;
#2319=ORIENTED_EDGE ( 'NONE', *, *, #2908, .T. ) ;
#2320=CARTESIAN_POINT ( 'NONE',  ( -57.08002265617300708, 84.22855780814606419, -15.00000000000000711 ) ) ;
#2321=CARTESIAN_POINT ( 'NONE',  ( -73.62877340657378511, 59.96410525291461369, 22.93460344427330000 ) ) ;
#2326=DIRECTION ( 'NONE',  ( -1.000000000000000000, 0.000000000000000000, -0.000000000000000000 ) ) ;
#2328=DIRECTION ( 'NONE',  ( -0.000000000000000000, 1.000000000000000000, 0.000000000000000000 ) ) ;
#2330=VERTEX_POINT ( 'NONE', #17199 ) ;
#2331=DIRECTION ( 'NONE',  ( -0.000000000000000000, 0.000000000000000000, -1.000000000000000000 ) ) ;
#2359=DIRECTION ( 'NONE',  ( -1.000000000000000000, -0.000000000000000000, -0.000000000000000000 ) ) ;
#2362=VERTEX_POINT ( 'NONE', #8872 ) ;
#2366=ORIENTED_EDGE ( 'NONE', *, *, #7655, .T. ) ;
#2367=DIRECTION ( 'NONE',  ( 4.124608743189000987E-16, -1.000000000000000000, 0.000000000000000000 ) ) ;
#2372=CARTESIAN_POINT ( 'NONE',  ( -75.30099397498476321, 107.2622484790587407, -24.10072931937693141 ) ) ;
#2390=AXIS2_PLACEMENT_3D ( 'NONE', #6723, #5310, #916 ) ;
#2391=DIRECTION ( 'NONE',  ( -0.000000000000000000, -0.000000000000000000, -1.000000000000000000 ) ) ;
#2429=ORIENTED_EDGE ( 'NONE', *, *, #9390, .T. ) ;
#2442=CARTESIAN_POINT ( 'NONE',  ( -123.4618227840623632, -151.5628872026273086, -57.00000000000000000 ) ) ;
#2445=CARTESIAN_POINT ( 'NONE',  ( -36.44155368744861079, 56.74635804676025685, 0.000000000000000000 ) ) ;
#2447=DIRECTION ( 'NONE',  ( -4.675871521838984962E-16, 1.000000000000000000, 0.000000000000000000 ) ) ;
#2451=CARTESIAN_POINT ( 'NONE',  ( -66.56242279005481066, 112.0249532631118399, 24.56082634672266707 ) ) ;
#2461=ORIENTED_EDGE ( 'NONE', *, *, #9720, .T. ) ;
#2463=EDGE_LOOP ( 'NONE', ( #12801, #6878, #9677, #17977 ) ) ;
#2464=VECTOR ( 'NONE', #14089, 1000.000000000000000 ) ;
#2466=CARTESIAN_POINT ( 'NONE',  ( 15.23320273812466041, -46.83756720124470263, 115.7605492041889619 ) ) ;
#2472=DIRECTION ( 'NONE',  ( -0.9475106458593564041, 0.3197242186372270534, -0.000000000000000000 ) ) ;
#2476=CARTESIAN_POINT ( 'NONE',  ( -66.63376473465912397, -19.34983604512935429, 57.00000000000000000 ) ) ;
#2481=ORIENTED_EDGE ( 'NONE', *, *, #414, .T. ) ;
#2494=FACE_OUTER_BOUND ( 'NONE', #12973, .T. ) ;
#2495=CARTESIAN_POINT ( 'NONE',  ( -57.08002265617300708, 84.22855780814606419, 25.00000000000000355 ) ) ;
#2497=CARTESIAN_POINT ( 'NONE',  ( -46.00604326503374608, 49.61971273109995195, 27.56969510706493764 ) ) ;
#2501=DIRECTION ( 'NONE',  ( 1.000000000000000000, 0.000000000000000000, 0.000000000000000000 ) ) ;
#2504=CARTESIAN_POINT ( 'NONE',  ( 4.873318353650091694, -11.10456963339436598, -53.31387177695791735 ) ) ;
#2506=ORIENTED_EDGE ( 'NONE', *, *, #17580, .F. ) ;
#2508=DIRECTION ( 'NONE',  ( -1.000000000000000000, -0.000000000000000000, -0.000000000000000000 ) ) ;
#2509=EDGE_CURVE ( 'NONE', #11177, #6138, #6980, .T. ) ;
#2515=DIRECTION ( 'NONE',  ( -1.000000000000000000, -4.124608743189000987E-16, 0.000000000000000000 ) ) ;
#2520=DIRECTION ( 'NONE',  ( -0.000000000000000000, -0.000000000000000000, 1.000000000000000000 ) ) ;
#2521=CARTESIAN_POINT ( 'NONE',  ( -66.34341644926747961, 56.84031775370380046, -27.99999999999999645 ) ) ;
#2524=EDGE_CURVE ( 'NONE', #15955, #11788, #13632, .T. ) ;
#2525=DIRECTION ( 'NONE',  ( 1.000000000000000000, 2.062304371594500494E-16, -0.000000000000000000 ) ) ;
#2544=EDGE_CURVE ( 'NONE', #6958, #8849, #1907, .T. ) ;
#2570=ORIENTED_EDGE ( 'NONE', *, *, #678, .F. ) ;
#2572=ORIENTED_EDGE ( 'NONE', *, *, #15789, .T. ) ;
#2573=VECTOR ( 'NONE', #1278, 1000.000000000000114 ) ;
#2575=DIRECTION ( 'NONE',  ( 0.000000000000000000, 0.000000000000000000, 1.000000000000000000 ) ) ;
#2579=CARTESIAN_POINT ( 'NONE',  ( -36.44155368744860368, 56.74635804676025685, -22.50216374311546019 ) ) ;
#2580=DIRECTION ( 'NONE',  ( -0.000000000000000000, 1.000000000000000000, 0.000000000000000000 ) ) ;
#2581=VERTEX_POINT ( 'NONE', #5001 ) ;
#2582=CARTESIAN_POINT ( 'NONE',  ( -57.08002265617300708, 84.22855780814606419, -47.49999999999999289 ) ) ;
#2584=DIRECTION ( 'NONE',  ( 0.000000000000000000, 0.000000000000000000, 1.000000000000000000 ) ) ;
#2595=DIRECTION ( 'NONE',  ( 0.000000000000000000, -1.000000000000000000, 0.000000000000000000 ) ) ;
#2607=FACE_OUTER_BOUND ( 'NONE', #13874, .T. ) ;
#2614=ORIENTED_EDGE ( 'NONE', *, *, #1969, .F. ) ;
#2618=DIRECTION ( 'NONE',  ( 0.000000000000000000, -1.000000000000000000, 0.000000000000000000 ) ) ;
#2619=DIRECTION ( 'NONE',  ( 1.000000000000000000, 2.062304371594500494E-16, -0.000000000000000000 ) ) ;
#2620=ORIENTED_EDGE ( 'NONE', *, *, #11343, .T. ) ;
#2632=ORIENTED_EDGE ( 'NONE', *, *, #15806, .T. ) ;
#2643=ORIENTED_EDGE ( 'NONE', *, *, #5496, .T. ) ;
#2651=EDGE_CURVE ( 'NONE', #8001, #17304, #2207, .T. ) ;
#2665=EDGE_CURVE ( 'NONE', #13490, #2052, #17722, .T. ) ;
#2669=DIRECTION ( 'NONE',  ( -0.000000000000000000, -0.000000000000000000, -1.000000000000000000 ) ) ;
#2673=EDGE_LOOP ( 'NONE', ( #4761, #12857, #12685, #17857, #9212 ) ) ;
#2676=CARTESIAN_POINT ( 'NONE',  ( -92.59262256747319952, 57.88796029049329661, 26.35917033480641436 ) ) ;
#2678=B_SPLINE_CURVE_WITH_KNOTS ( 'NONE', 3,
 ( #5562, #5465, #13995, #1175 ),
 .UNSPECIFIED., .F., .F.,
 ( 4, 4 ),
 ( 0.007714237994431366770, 0.01042320952183839987 ),
 .UNSPECIFIED. ) ;
#2683=LINE ( 'NONE', #8202, #17588 ) ;
#2684=DIRECTION ( 'NONE',  ( -0.000000000000000000, -0.000000000000000000, -1.000000000000000000 ) ) ;
#2706=EDGE_CURVE ( 'NONE', #9223, #4742, #10864, .T. ) ;
#2709=CARTESIAN_POINT ( 'NONE',  ( 95.45835937779679625, 56.41207303426869402, 7.000000000000010658 ) ) ;
#2710=CARTESIAN_POINT ( 'NONE',  ( -92.59262256747321373, 110.5691553257988460, 26.35917033480641436 ) ) ;
#2713=CARTESIAN_POINT ( 'NONE',  ( -66.85187407874441590, 108.3380026262840090, -27.99999999999999645 ) ) ;
#2714=LINE ( 'NONE', #1038, #14992 ) ;
#2721=DIRECTION ( 'NONE',  ( -1.000000000000000000, -0.000000000000000000, -0.000000000000000000 ) ) ;
#2728=VECTOR ( 'NONE', #13517, 1000.000000000000000 ) ;
#2729=CARTESIAN_POINT ( 'NONE',  ( -67.59262256747317110, 56.80567558672318995, -22.50837044127973030 ) ) ;
#2739=FACE_OUTER_BOUND ( 'NONE', #17231, .T. ) ;
#2740=CARTESIAN_POINT ( 'NONE',  ( 105.4583593777967963, -32.62665103886256190, 7.000000000000010658 ) ) ;
#2756=CIRCLE ( 'NONE', #9624, 3.999999999999982681 ) ;
#2758=VECTOR ( 'NONE', #4406, 1000.000000000000000 ) ;
#2759=CARTESIAN_POINT ( 'NONE',  ( 7.757986314337494527, 14.88675170491334221, -45.60895101101229443 ) ) ;
#2760=CARTESIAN_POINT ( 'NONE',  ( -57.08002265617300708, 84.22855780814606419, -35.00000000000000711 ) ) ;
#2764=CARTESIAN_POINT ( 'NONE',  ( 124.5381772159375942, -151.5628872026272802, 57.00000000000000000 ) ) ;
#2765=ORIENTED_EDGE ( 'NONE', *, *, #16546, .F. ) ;
#2768=VERTEX_POINT ( 'NONE', #10241 ) ;
#2769=ADVANCED_FACE ( 'NONE', ( #6107 ), #15854, .F. ) ;
#2775=AXIS2_PLACEMENT_3D ( 'NONE', #11927, #10522, #14821 ) ;
#2777=ORIENTED_EDGE ( 'NONE', *, *, #6152, .T. ) ;
#2779=ADVANCED_FACE ( 'NONE', ( #4363 ), #10068, .T. ) ;
#2787=CARTESIAN_POINT ( 'NONE',  ( -57.08002265617300708, 84.22855780814606419, 28.00000000000000355 ) ) ;
#2788=DIRECTION ( 'NONE',  ( 1.000000000000000000, 0.000000000000000000, 0.000000000000000000 ) ) ;
#2794=VECTOR ( 'NONE', #12786, 1000.000000000000000 ) ;
#2800=VECTOR ( 'NONE', #9652, 1000.000000000000000 ) ;
#2809=VERTEX_POINT ( 'NONE', #3685 ) ;
#2811=CARTESIAN_POINT ( 'NONE',  ( -68.43628269749412141, 111.3280217493016266, -22.41747227276117727 ) ) ;
#2814=CARTESIAN_POINT ( 'NONE',  ( -66.20572860746047184, 111.1782190889722983, -28.00000000000000355 ) ) ;
#2816=CARTESIAN_POINT ( 'NONE',  ( 124.5381772159375942, -111.0842361345572158, 57.00000000000000000 ) ) ;
#2819=( GEOMETRIC_REPRESENTATION_CONTEXT ( 3 ) GLOBAL_UNCERTAINTY_ASSIGNED_CONTEXT ( ( #16559 ) ) GLOBAL_UNIT_ASSIGNED_CONTEXT ( ( #443, #14568, #5870 ) ) REPRESENTATION_CONTEXT ( 'NONE', 'WORKASPACE' ) );
#2824=DIRECTION ( 'NONE',  ( 0.000000000000000000, 0.000000000000000000, 1.000000000000000000 ) ) ;
#2835=CARTESIAN_POINT ( 'NONE',  ( -67.59262256747317110, 61.53592931583062153, -28.00000000000000355 ) ) ;
#2841=ORIENTED_EDGE ( 'NONE', *, *, #16008, .F. ) ;
#2848=VECTOR ( 'NONE', #8624, 1000.000000000000000 ) ;
#2858=CARTESIAN_POINT ( 'NONE',  ( 14.89901151198486495, -10.87016367198019040, -53.26726757078508712 ) ) ;
#2861=CARTESIAN_POINT ( 'NONE',  ( -57.08002265617300708, 84.22855780814606419, -28.00000000000000355 ) ) ;
#2865=ORIENTED_EDGE ( 'NONE', *, *, #15817, .F. ) ;
#2870=VECTOR ( 'NONE', #17921, 1000.000000000000000 ) ;
#2879=CARTESIAN_POINT ( 'NONE',  ( -67.59262256747317110, 57.88796029049329661, 26.35917033480641436 ) ) ;
#2888=CARTESIAN_POINT ( 'NONE',  ( 10.78766931562283737, 7.280728192202457372, 48.30793737034424140 ) ) ;
#2902=CARTESIAN_POINT ( 'NONE',  ( -67.59262256747319952, 111.6514400295689171, -22.50837044127971254 ) ) ;
#2903=DIRECTION ( 'NONE',  ( 0.000000000000000000, 0.000000000000000000, 1.000000000000000000 ) ) ;
#2906=LINE ( 'NONE', #8526, #4764 ) ;
#2908=EDGE_CURVE ( 'NONE', #14911, #6285, #14073, .T. ) ;
#2919=CARTESIAN_POINT ( 'NONE',  ( -50.06979403241811610, 50.58224449241410525, 57.00000000000000000 ) ) ;
#2921=LINE ( 'NONE', #3007, #3548 ) ;
#2927=CARTESIAN_POINT ( 'NONE',  ( -50.41499038512538533, 117.9449492212793444, -2.999999999999999112 ) ) ;
#2932=EDGE_CURVE ( 'NONE', #13980, #13829, #15051, .T. ) ;
#2937=ORIENTED_EDGE ( 'NONE', *, *, #9273, .T. ) ;
#2942=AXIS2_PLACEMENT_3D ( 'NONE', #11171, #6954, #18378 ) ;
#2948=ORIENTED_EDGE ( 'NONE', *, *, #416, .T. ) ;
#2952=ORIENTED_EDGE ( 'NONE', *, *, #18454, .F. ) ;
#2953=VERTEX_POINT ( 'NONE', #17319 ) ;
#2954=CARTESIAN_POINT ( 'NONE',  ( -57.08002265617300708, 84.22855780814606419, 28.00000000000000355 ) ) ;
#2956=ORIENTED_EDGE ( 'NONE', *, *, #1640, .T. ) ;
#2961=ORIENTED_EDGE ( 'NONE', *, *, #14484, .T. ) ;
#2966=CARTESIAN_POINT ( 'NONE',  ( -67.59262256747315689, 117.8748711238780373, 35.00000000000000000 ) ) ;
#2973=ORIENTED_EDGE ( 'NONE', *, *, #3549, .F. ) ;
#2979=CARTESIAN_POINT ( 'NONE',  ( -66.34428321731556366, 112.0980243198733177, -27.54384358185309267 ) ) ;
#2981=CARTESIAN_POINT ( 'NONE',  ( -70.06856178257680767, 110.5691553257988460, -22.35917033480641791 ) ) ;
#2983=EDGE_CURVE ( 'NONE', #13683, #11287, #11624, .T. ) ;
#2987=CARTESIAN_POINT ( 'NONE',  ( -39.99251679397033854, 54.40212825384665507, 24.22832327945725339 ) ) ;
#2997=ORIENTED_EDGE ( 'NONE', *, *, #13144, .T. ) ;
#3005=FACE_OUTER_BOUND ( 'NONE', #18345, .T. ) ;
#3007=CARTESIAN_POINT ( 'NONE',  ( -27.71117476891160081, 84.22855780814606419, 37.50000000000000000 ) ) ;
#3010=AXIS2_PLACEMENT_3D ( 'NONE', #1602, #16165, #8897 ) ;
#3017=CARTESIAN_POINT ( 'NONE',  ( 103.5381772159376084, -151.5628872026272802, -57.00000000000000000 ) ) ;
#3021=CIRCLE ( 'NONE', #5401, 29.36884788726140627 ) ;
#3032=DIRECTION ( 'NONE',  ( 0.000000000000000000, -1.000000000000000000, 0.000000000000000000 ) ) ;
#3035=ORIENTED_EDGE ( 'NONE', *, *, #13624, .F. ) ;
#3044=LINE ( 'NONE', #14284, #14457 ) ;
#3055=VERTEX_POINT ( 'NONE', #18472 ) ;
#3056=CIRCLE ( 'NONE', #6627, 3.999999999999982681 ) ;
#3057=VECTOR ( 'NONE', #7463, 1000.000000000000000 ) ;
#3060=VERTEX_POINT ( 'NONE', #5991 ) ;
#3066=AXIS2_PLACEMENT_3D ( 'NONE', #6000, #14705, #1634 ) ;
#3069=DIRECTION ( 'NONE',  ( -1.000000000000000000, 0.000000000000000000, 0.000000000000000000 ) ) ;
#3070=DIRECTION ( 'NONE',  ( 0.000000000000000000, 1.000000000000000000, -0.000000000000000000 ) ) ;
#3081=ORIENTED_EDGE ( 'NONE', *, *, #331, .T. ) ;
#3088=VERTEX_POINT ( 'NONE', #1792 ) ;
#3089=EDGE_CURVE ( 'NONE', #8537, #16154, #12776, .T. ) ;
#3097=EDGE_CURVE ( 'NONE', #3566, #3387, #8198, .T. ) ;
#3100=FACE_OUTER_BOUND ( 'NONE', #11232, .T. ) ;
#3101=ORIENTED_EDGE ( 'NONE', *, *, #11657, .T. ) ;
#3102=ADVANCED_FACE ( 'NONE', ( #17507, #7500 ), #3375, .F. ) ;
#3110=DIRECTION ( 'NONE',  ( 1.000000000000000000, 1.890137176791858990E-15, 0.000000000000000000 ) ) ;
#3111=VERTEX_POINT ( 'NONE', #9190 ) ;
#3119=DIRECTION ( 'NONE',  ( -0.000000000000000000, -0.000000000000000000, -1.000000000000000000 ) ) ;
#3129=CARTESIAN_POINT ( 'NONE',  ( -92.59262256747321373, 110.5691553257988460, 22.35917033480641791 ) ) ;
#3130=LINE ( 'NONE', #15760, #9344 ) ;
#3137=ORIENTED_EDGE ( 'NONE', *, *, #15912, .T. ) ;
#3143=FACE_OUTER_BOUND ( 'NONE', #16817, .T. ) ;
#3160=ORIENTED_EDGE ( 'NONE', *, *, #3423, .T. ) ;
#3163=DIRECTION ( 'NONE',  ( 0.000000000000000000, 1.245108978942215720E-14, 1.000000000000000000 ) ) ;
#3169=LINE ( 'NONE', #12049, #10628 ) ;
#3175=CARTESIAN_POINT ( 'NONE',  ( -66.09688823571623573, 58.56582669723388790, 25.00000000000000711 ) ) ;
#3182=DIRECTION ( 'NONE',  ( -0.000000000000000000, -0.000000000000000000, -1.000000000000000000 ) ) ;
#3185=DIRECTION ( 'NONE',  ( -1.000000000000000000, -0.000000000000000000, -0.000000000000000000 ) ) ;
#3187=VERTEX_POINT ( 'NONE', #17784 ) ;
#3188=DIRECTION ( 'NONE',  ( 1.000000000000000000, 0.000000000000000000, 5.204170427930409450E-16 ) ) ;
#3189=EDGE_CURVE ( 'NONE', #4169, #1925, #6402, .T. ) ;
#3195=EDGE_LOOP ( 'NONE', ( #17452, #9590, #17464, #18351 ) ) ;
#3208=EDGE_CURVE ( 'NONE', #8420, #9318, #18050, .T. ) ;
#3209=CARTESIAN_POINT ( 'NONE',  ( -57.08002265617300708, 84.22855780814606419, 37.50000000000000000 ) ) ;
#3210=ADVANCED_FACE ( 'NONE', ( #10965 ), #15455, .F. ) ;
#3213=VERTEX_POINT ( 'NONE', #9651 ) ;
#3247=PLANE ( 'NONE',  #7636 ) ;
#3253=CARTESIAN_POINT ( 'NONE',  ( -67.25653033657522428, 61.05141432888216713, 25.00000000000000355 ) ) ;
#3275=CARTESIAN_POINT ( 'NONE',  ( 105.4583593777968105, 56.41207303426870112, -7.000000000000010658 ) ) ;
#3279=ORIENTED_EDGE ( 'NONE', *, *, #5010, .F. ) ;
#3287=DIRECTION ( 'NONE',  ( 1.000000000000000000, 2.062304371594500494E-16, -0.000000000000000000 ) ) ;
#3309=VERTEX_POINT ( 'NONE', #10868 ) ;
#3315=ORIENTED_EDGE ( 'NONE', *, *, #10863, .T. ) ;
#3326=ORIENTED_EDGE ( 'NONE', *, *, #5172, .T. ) ;
#3331=CARTESIAN_POINT ( 'NONE',  ( -92.59262256747319952, 57.88796029049329661, -30.35917033480640370 ) ) ;
#3335=AXIS2_PLACEMENT_3D ( 'NONE', #3437, #3338, #9153 ) ;
#3338=DIRECTION ( 'NONE',  ( -1.000000000000000000, -0.000000000000000000, -0.000000000000000000 ) ) ;
#3344=VECTOR ( 'NONE', #12777, 1000.000000000000000 ) ;
#3345=LINE ( 'NONE', #13279, #15243 ) ;
#3350=VECTOR ( 'NONE', #16574, 1000.000000000000000 ) ;
#3352=DIRECTION ( 'NONE',  ( 0.000000000000000000, -1.000000000000000000, 0.000000000000000000 ) ) ;
#3359=ORIENTED_EDGE ( 'NONE', *, *, #5390, .F. ) ;
#3375=PLANE ( 'NONE',  #14467 ) ;
#3387=VERTEX_POINT ( 'NONE', #11437 ) ;
#3389=LINE ( 'NONE', #588, #4146 ) ;
#3404=EDGE_LOOP ( 'NONE', ( #13761, #17961, #6229, #8779, #13764 ) ) ;
#3408=FACE_BOUND ( 'NONE', #11172, .T. ) ;
#3414=AXIS2_PLACEMENT_3D ( 'NONE', #4159, #5461, #14082 ) ;
#3418=EDGE_CURVE ( 'NONE', #10351, #13411, #5889, .T. ) ;
#3419=ORIENTED_EDGE ( 'NONE', *, *, #4942, .T. ) ;
#3423=EDGE_CURVE ( 'NONE', #5426, #14435, #2921, .T. ) ;
#3434=CARTESIAN_POINT ( 'NONE',  ( -57.08002265617300708, 84.22855780814606419, 37.50000000000000000 ) ) ;
#3436=VECTOR ( 'NONE', #13841, 1000.000000000000000 ) ;
#3437=CARTESIAN_POINT ( 'NONE',  ( -67.59262256747319952, 110.5691553257988460, -26.35917033480641436 ) ) ;
#3438=CARTESIAN_POINT ( 'NONE',  ( -66.00585202009801833, 57.88796029049324687, 25.00000000000000355 ) ) ;
#3440=ADVANCED_FACE ( 'NONE', ( #203 ), #7050, .F. ) ;
#3449=ORIENTED_EDGE ( 'NONE', *, *, #10923, .F. ) ;
#3470=LINE ( 'NONE', #1785, #16081 ) ;
#3472=VERTEX_POINT ( 'NONE', #15997 ) ;
#3488=ORIENTED_EDGE ( 'NONE', *, *, #8590, .T. ) ;
#3490=VERTEX_POINT ( 'NONE', #9424 ) ;
#3501=VERTEX_POINT ( 'NONE', #4668 ) ;
#3502=DIRECTION ( 'NONE',  ( 0.000000000000000000, 0.000000000000000000, 1.000000000000000000 ) ) ;
#3507=ORIENTED_EDGE ( 'NONE', *, *, #14030, .F. ) ;
#3512=EDGE_CURVE ( 'NONE', #15291, #17238, #1771, .T. ) ;
#3517=DIRECTION ( 'NONE',  ( 2.062304371594500494E-16, -1.000000000000000000, 0.000000000000000000 ) ) ;
#3520=VECTOR ( 'NONE', #1205, 1000.000000000000000 ) ;
#3526=ORIENTED_EDGE ( 'NONE', *, *, #11566, .T. ) ;
#3528=CARTESIAN_POINT ( 'NONE',  ( 95.45835937779683888, -32.62665103886254059, 7.000000000000010658 ) ) ;
#3529=DIRECTION ( 'NONE',  ( -1.000000000000000000, -0.000000000000000000, -0.000000000000000000 ) ) ;
#3542=DIRECTION ( 'NONE',  ( 1.000000000000000000, 0.000000000000000000, 0.000000000000000000 ) ) ;
#3545=EDGE_CURVE ( 'NONE', #18444, #4298, #12618, .T. ) ;
#3546=CARTESIAN_POINT ( 'NONE',  ( -75.16379081051663036, 61.08681906830677377, -23.95122000524899164 ) ) ;
#3548=VECTOR ( 'NONE', #14420, 1000.000000000000000 ) ;
#3549=EDGE_CURVE ( 'NONE', #8849, #14752, #4178, .T. ) ;
#3550=ORIENTED_EDGE ( 'NONE', *, *, #13648, .F. ) ;
#3555=ORIENTED_EDGE ( 'NONE', *, *, #6780, .T. ) ;
#3557=DIRECTION ( 'NONE',  ( -1.000000000000000000, -0.000000000000000000, -0.000000000000000000 ) ) ;
#3566=VERTEX_POINT ( 'NONE', #17086 ) ;
#3575=ORIENTED_EDGE ( 'NONE', *, *, #10532, .T. ) ;
#3578=ORIENTED_EDGE ( 'NONE', *, *, #244, .F. ) ;
#3590=FACE_BOUND ( 'NONE', #12304, .T. ) ;
#3597=VECTOR ( 'NONE', #426, 1000.000000000000000 ) ;
#3599=DIRECTION ( 'NONE',  ( -0.000000000000000000, -0.000000000000000000, -1.000000000000000000 ) ) ;
#3605=CARTESIAN_POINT ( 'NONE',  ( -64.09025127992791226, 117.8748711238780373, 7.000000000000009770 ) ) ;
#3618=DIRECTION ( 'NONE',  ( -0.000000000000000000, -0.000000000000000000, -1.000000000000000000 ) ) ;
#3625=VECTOR ( 'NONE', #16749, 1000.000000000000000 ) ;
#3630=DIRECTION ( 'NONE',  ( -1.000000000000000000, -0.000000000000000000, -0.000000000000000000 ) ) ;
#3638=DIRECTION ( 'NONE',  ( 0.000000000000000000, 0.000000000000000000, -1.000000000000000000 ) ) ;
#3639=DIRECTION ( 'NONE',  ( 1.000000000000000000, 1.119176436114069332E-16, 0.000000000000000000 ) ) ;
#3666=CARTESIAN_POINT ( 'NONE',  ( -67.15882256147138207, 111.8146619846916821, 23.31672727879027462 ) ) ;
#3668=CARTESIAN_POINT ( 'NONE',  ( -70.71978124295696944, -111.0842361345572158, -18.23991632971910803 ) ) ;
#3669=LINE ( 'NONE', #7695, #3350 ) ;
#3672=EDGE_LOOP ( 'NONE', ( #5389, #609, #2643, #3697 ) ) ;
#3675=EDGE_CURVE ( 'NONE', #4742, #7351, #16088, .T. ) ;
#3685=CARTESIAN_POINT ( 'NONE',  ( -92.59262256747321373, 110.5691553257988460, -22.35917033480641791 ) ) ;
#3696=AXIS2_PLACEMENT_3D ( 'NONE', #4921, #9141, #9502 ) ;
#3697=ORIENTED_EDGE ( 'NONE', *, *, #14225, .T. ) ;
#3698=AXIS2_PLACEMENT_3D ( 'NONE', #2954, #14364, #14461 ) ;
#3700=CARTESIAN_POINT ( 'NONE',  ( -66.31963392321378592, 109.2426495258444277, 25.00000000000000355 ) ) ;
#3715=CARTESIAN_POINT ( 'NONE',  ( -1.861400446476476622, 12.03450721920232880, 46.70170638485993919 ) ) ;
#3721=CARTESIAN_POINT ( 'NONE',  ( -24.54889247506734762, 50.87908043791564694, 26.71068393001068131 ) ) ;
#3740=CARTESIAN_POINT ( 'NONE',  ( -73.11430033901579861, 59.62110470154726016, 22.74887301420309882 ) ) ;
#3743=DIRECTION ( 'NONE',  ( -0.000000000000000000, -0.000000000000000000, 1.000000000000000000 ) ) ;
#3748=FACE_OUTER_BOUND ( 'NONE', #3761, .T. ) ;
#3761=EDGE_LOOP ( 'NONE', ( #9423, #12681, #13215, #16201 ) ) ;
#3764=DIRECTION ( 'NONE',  ( -1.000000000000000000, -2.826528109797569363E-15, 0.000000000000000000 ) ) ;
#3772=ADVANCED_FACE ( 'NONE', ( #16036 ), #17182, .F. ) ;
#3788=CARTESIAN_POINT ( 'NONE',  ( -75.16338607169024044, 107.3706141836132986, -23.95078896739801522 ) ) ;
#3789=CARTESIAN_POINT ( 'NONE',  ( -66.02576182061889654, 110.2283017972794141, 25.00000000000000711 ) ) ;
#3790=ORIENTED_EDGE ( 'NONE', *, *, #255, .F. ) ;
#3793=CARTESIAN_POINT ( 'NONE',  ( -123.4618227840623632, -151.5628872026273086, -57.00000000000000000 ) ) ;
#3802=ORIENTED_EDGE ( 'NONE', *, *, #13172, .F. ) ;
#3806=CARTESIAN_POINT ( 'NONE',  ( -57.08002265617300708, 84.22855780814606419, 25.00000000000000355 ) ) ;
#3812=CARTESIAN_POINT ( 'NONE',  ( -21.11045101004114599, 48.70050140195975530, 28.18094419443968235 ) ) ;
#3815=LINE ( 'NONE', #5114, #5971 ) ;
#3820=CARTESIAN_POINT ( 'NONE',  ( -57.08002265617300708, 84.22855780814606419, -2.999999999999999112 ) ) ;
#3822=DIRECTION ( 'NONE',  ( 0.000000000000000000, -4.000800291689476871E-17, -1.000000000000000000 ) ) ;
#3829=LINE ( 'NONE', #9824, #9625 ) ;
#3852=FACE_OUTER_BOUND ( 'NONE', #10007, .T. ) ;
#3856=ORIENTED_EDGE ( 'NONE', *, *, #8372, .F. ) ;
#3858=EDGE_CURVE ( 'NONE', #9128, #8646, #7451, .T. ) ;
#3861=CIRCLE ( 'NONE', #4787, 26.04359719766049608 ) ;
#3864=CARTESIAN_POINT ( 'NONE',  ( -102.4618227840623774, 0.000000000000000000, 36.00000000000000711 ) ) ;
#3871=DIRECTION ( 'NONE',  ( -1.000000000000000000, 0.000000000000000000, 0.000000000000000000 ) ) ;
#3872=DIRECTION ( 'NONE',  ( -0.000000000000000000, -0.000000000000000000, 1.000000000000000000 ) ) ;
#3882=EDGE_CURVE ( 'NONE', #3060, #14435, #7171, .T. ) ;
#3891=VECTOR ( 'NONE', #14043, 1000.000000000000000 ) ;
#3894=DIRECTION ( 'NONE',  ( -0.000000000000000000, -0.000000000000000000, 1.000000000000000000 ) ) ;
#3901=CARTESIAN_POINT ( 'NONE',  ( -5.341607757298564074, 34.93162786869717706, 36.42599446819355791 ) ) ;
#3909=LINE ( 'NONE', #12733, #11929 ) ;
#3911=ORIENTED_EDGE ( 'NONE', *, *, #15912, .F. ) ;
#3913=ORIENTED_EDGE ( 'NONE', *, *, #2524, .F. ) ;
#3916=ORIENTED_EDGE ( 'NONE', *, *, #5236, .F. ) ;
#3919=CARTESIAN_POINT ( 'NONE',  ( -66.20510745737880143, 58.30955781107306279, -28.00000000000000355 ) ) ;
#3920=PLANE ( 'NONE',  #5070 ) ;
#3922=DIRECTION ( 'NONE',  ( 0.000000000000000000, 0.000000000000000000, 1.000000000000000000 ) ) ;
#3923=CARTESIAN_POINT ( 'NONE',  ( -36.44155368744862500, 56.74635804676027107, -2.999999999999999112 ) ) ;
#3925=EDGE_CURVE ( 'NONE', #6726, #3490, #16396, .T. ) ;
#3928=ORIENTED_EDGE ( 'NONE', *, *, #15817, .T. ) ;
#3936=VERTEX_POINT ( 'NONE', #10996 ) ;
#3939=DIRECTION ( 'NONE',  ( 0.000000000000000000, 0.000000000000000000, 1.000000000000000000 ) ) ;
#3947=CARTESIAN_POINT ( 'NONE',  ( -92.59262256747319952, 50.58224449241410525, 15.00000000000005862 ) ) ;
#3955=VERTEX_POINT ( 'NONE', #12506 ) ;
#3968=CARTESIAN_POINT ( 'NONE',  ( -57.08002265617300708, 84.22855780814606419, 37.50000000000000000 ) ) ;
#3972=CARTESIAN_POINT ( 'NONE',  ( -76.14791583990366064, 106.5656527319057147, -26.51439991379068672 ) ) ;
#3975=AXIS2_PLACEMENT_3D ( 'NONE', #12078, #13301, #3638 ) ;
#3978=CARTESIAN_POINT ( 'NONE',  ( -66.13756031549399950, 56.29129655451910708, -26.34212773717771583 ) ) ;
#3979=ORIENTED_EDGE ( 'NONE', *, *, #16236, .F. ) ;
#3993=DIRECTION ( 'NONE',  ( -1.000000000000000000, 0.000000000000000000, 0.000000000000000000 ) ) ;
#3996=CARTESIAN_POINT ( 'NONE',  ( -100.4870060002411805, -151.5628872026273086, 57.00000000000000000 ) ) ;
#3998=( LENGTH_UNIT ( ) NAMED_UNIT ( * ) SI_UNIT ( .MILLI., .METRE. ) );
#4003=AXIS2_PLACEMENT_3D ( 'NONE', #11482, #4702, #234 ) ;
#4016=DIRECTION ( 'NONE',  ( -0.000000000000000000, -0.000000000000000000, -1.000000000000000000 ) ) ;
#4018=CARTESIAN_POINT ( 'NONE',  ( -67.59262256747317110, 56.80567558672318995, 22.50837044127973030 ) ) ;
#4028=DIRECTION ( 'NONE',  ( 0.000000000000000000, -1.000000000000000000, 4.000800291689476254E-17 ) ) ;
#4037=B_SPLINE_CURVE_WITH_KNOTS ( 'NONE', 3,
 ( #13562, #11138, #11035, #5128, #752, #6631, #12540, #16829 ),
 .UNSPECIFIED., .F., .F.,
 ( 4, 2, 2, 4 ),
 ( 0.01670317819300424014, 0.01709299363389421220, 0.01748280907478418772, 0.01826243995656414570 ),
 .UNSPECIFIED. ) ;
#4046=EDGE_CURVE ( 'NONE', #3566, #10531, #17246, .T. ) ;
#4049=ORIENTED_EDGE ( 'NONE', *, *, #15900, .T. ) ;
#4073=VERTEX_POINT ( 'NONE', #8570 ) ;
#4077=LINE ( 'NONE', #11085, #6590 ) ;
#4079=CARTESIAN_POINT ( 'NONE',  ( 5.233202738124664855, -111.0842361345572158, 57.00000000000000000 ) ) ;
#4092=CARTESIAN_POINT ( 'NONE',  ( -127.5926225674731995, 47.87487112387803023, -15.00000000000000355 ) ) ;
#4099=CARTESIAN_POINT ( 'NONE',  ( -75.58277579834157223, 107.0370988044063267, 24.46269018718348320 ) ) ;
#4100=CARTESIAN_POINT ( 'NONE',  ( -7.851504758905779369, 22.18492356653273134, -42.64945817991924315 ) ) ;
#4108=ORIENTED_EDGE ( 'NONE', *, *, #3882, .T. ) ;
#4109=EDGE_CURVE ( 'NONE', #16062, #13980, #4884, .T. ) ;
#4110=CARTESIAN_POINT ( 'NONE',  ( 0.000000000000000000, 0.000000000000000000, -35.00000000000000000 ) ) ;
#4111=ORIENTED_EDGE ( 'NONE', *, *, #2509, .F. ) ;
#4116=CARTESIAN_POINT ( 'NONE',  ( -92.59262256747321373, 110.5691553257988460, -26.35917033480641436 ) ) ;
#4124=EDGE_LOOP ( 'NONE', ( #15387, #18264, #3790, #1957, #16386, #17845 ) ) ;
#4140=CARTESIAN_POINT ( 'NONE',  ( -194.4437806548868934, -111.0842361345572158, 18.23991632971911869 ) ) ;
#4146=VECTOR ( 'NONE', #2176, 1000.000000000000000 ) ;
#4149=ORIENTED_EDGE ( 'NONE', *, *, #1063, .F. ) ;
#4158=CARTESIAN_POINT ( 'NONE',  ( -24.58056302216690625, 50.89799459937560755, -26.69769766716196457 ) ) ;
#4159=CARTESIAN_POINT ( 'NONE',  ( 103.5381772159376084, -111.0842361345572158, 36.00000000000000711 ) ) ;
#4160=ORIENTED_EDGE ( 'NONE', *, *, #10891, .F. ) ;
#4162=PLANE ( 'NONE',  #7803 ) ;
#4169=VERTEX_POINT ( 'NONE', #14707 ) ;
#4177=CARTESIAN_POINT ( 'NONE',  ( -57.08002265617300708, 84.22855780814606419, -47.49999999999999289 ) ) ;
#4178=LINE ( 'NONE', #14203, #2058 ) ;
#4188=VERTEX_POINT ( 'NONE', #7697 ) ;
#4197=VECTOR ( 'NONE', #8219, 1000.000000000000000 ) ;
#4228=CARTESIAN_POINT ( 'NONE',  ( -36.44155368744861079, 56.74635804676026396, 22.50216374311547440 ) ) ;
#4229=EDGE_LOOP ( 'NONE', ( #16511, #1531, #15557, #3137, #14602, #4397, #12872, #17375, #14562 ) ) ;
#4242=EDGE_CURVE ( 'NONE', #17405, #6830, #13880, .T. ) ;
#4243=CIRCLE ( 'NONE', #8736, 180.8515291679561585 ) ;
#4245=DIRECTION ( 'NONE',  ( -0.9475106458593564041, -0.3197242186372270534, -0.000000000000000000 ) ) ;
#4257=CARTESIAN_POINT ( 'NONE',  ( -64.09025127992791226, 109.3109350805793270, 37.50000000000000000 ) ) ;
#4260=EDGE_CURVE ( 'NONE', #12660, #505, #8063, .T. ) ;
#4261=B_SPLINE_CURVE_WITH_KNOTS ( 'NONE', 3,
 ( #8261, #18170, #3666, #16653, #2451, #14975 ),
 .UNSPECIFIED., .F., .F.,
 ( 4, 2, 4 ),
 ( 0.0004789955798651479406, 0.001874570251607515087, 0.003270144923349882233 ),
 .UNSPECIFIED. ) ;
#4287=CARTESIAN_POINT ( 'NONE',  ( -3.386515864108431195, 32.64046595754329161, 37.63508979505212437 ) ) ;
#4298=VERTEX_POINT ( 'NONE', #6851 ) ;
#4301=CARTESIAN_POINT ( 'NONE',  ( -123.4618227840623632, -151.5628872026273086, 57.00000000000000000 ) ) ;
#4325=DIRECTION ( 'NONE',  ( -1.000000000000000000, 0.000000000000000000, 0.000000000000000000 ) ) ;
#4328=DIRECTION ( 'NONE',  ( -1.000000000000000000, 1.558623840612994987E-16, 0.000000000000000000 ) ) ;
#4329=ORIENTED_EDGE ( 'NONE', *, *, #5149, .F. ) ;
#4330=AXIS2_PLACEMENT_3D ( 'NONE', #611, #9041, #2106 ) ;
#4331=AXIS2_PLACEMENT_3D ( 'NONE', #9404, #17716, #6480 ) ;
#4342=VECTOR ( 'NONE', #10748, 1000.000000000000000 ) ;
#4352=VERTEX_POINT ( 'NONE', #14062 ) ;
#4355=LINE ( 'NONE', #10064, #9697 ) ;
#4362=FACE_OUTER_BOUND ( 'NONE', #4813, .T. ) ;
#4363=FACE_OUTER_BOUND ( 'NONE', #17420, .T. ) ;
#4381=ORIENTED_EDGE ( 'NONE', *, *, #14548, .T. ) ;
#4382=ORIENTED_EDGE ( 'NONE', *, *, #5830, .F. ) ;
#4387=LINE ( 'NONE', #10095, #2800 ) ;
#4390=DIRECTION ( 'NONE',  ( 0.3197242186372270534, 0.9475106458593564041, 0.000000000000000000 ) ) ;
#4395=DIRECTION ( 'NONE',  ( 1.000000000000000000, 1.119176436114069332E-16, 0.000000000000000000 ) ) ;
#4397=ORIENTED_EDGE ( 'NONE', *, *, #1407, .F. ) ;
#4406=DIRECTION ( 'NONE',  ( -0.000000000000000000, -0.000000000000000000, 1.000000000000000000 ) ) ;
#4410=EDGE_CURVE ( 'NONE', #18251, #2177, #12678, .T. ) ;
#4424=DIRECTION ( 'NONE',  ( 0.000000000000000000, 0.000000000000000000, -1.000000000000000000 ) ) ;
#4432=AXIS2_PLACEMENT_3D ( 'NONE', #8905, #1884, #390 ) ;
#4436=DIRECTION ( 'NONE',  ( 0.000000000000000000, 0.000000000000000000, 1.000000000000000000 ) ) ;
#4439=DIRECTION ( 'NONE',  ( 1.000000000000000000, 0.000000000000000000, 0.000000000000000000 ) ) ;
#4454=ORIENTED_EDGE ( 'NONE', *, *, #17262, .T. ) ;
#4460=ADVANCED_FACE ( 'NONE', ( #12770 ), #17140, .F. ) ;
#4464=ADVANCED_FACE ( 'NONE', ( #5814 ), #15550, .T. ) ;
#4466=VERTEX_POINT ( 'NONE', #10043 ) ;
#4471=ORIENTED_EDGE ( 'NONE', *, *, #11817, .F. ) ;
#4482=VERTEX_POINT ( 'NONE', #481 ) ;
#4492=CARTESIAN_POINT ( 'NONE',  ( 5.233202738124664855, -19.34983604512935074, 57.00000000000000000 ) ) ;
#4506=DIRECTION ( 'NONE',  ( 0.000000000000000000, 0.000000000000000000, -1.000000000000000000 ) ) ;
#4507=B_SPLINE_CURVE_WITH_KNOTS ( 'NONE', 3,
 ( #12351, #9627, #927, #11238, #1029, #4018 ),
 .UNSPECIFIED., .F., .F.,
 ( 4, 2, 4 ),
 ( 0.0002781749886595805371, 0.001673372216920096913, 0.003068569445180613017 ),
 .UNSPECIFIED. ) ;
#4512=ORIENTED_EDGE ( 'NONE', *, *, #16946, .T. ) ;
#4524=VECTOR ( 'NONE', #16570, 1000.000000000000000 ) ;
#4527=ORIENTED_EDGE ( 'NONE', *, *, #18318, .F. ) ;
#4538=CIRCLE ( 'NONE', #1849, 34.36884788726141693 ) ;
#4543=VERTEX_POINT ( 'NONE', #17401 ) ;
#4544=ORIENTED_EDGE ( 'NONE', *, *, #17224, .T. ) ;
#4546=ORIENTED_EDGE ( 'NONE', *, *, #9609, .F. ) ;
#4552=CARTESIAN_POINT ( 'NONE',  ( -70.06856178257687873, 57.88796029049330372, -22.35917033480642502 ) ) ;
#4568=CARTESIAN_POINT ( 'NONE',  ( -66.00585202009860097, 58.06035137085946474, 25.00000000000000000 ) ) ;
#4575=VERTEX_POINT ( 'NONE', #10579 ) ;
#4583=DIRECTION ( 'NONE',  ( 0.000000000000000000, -1.000000000000000000, 0.000000000000000000 ) ) ;
#4594=DIRECTION ( 'NONE',  ( 0.000000000000000000, 0.000000000000000000, 1.000000000000000000 ) ) ;
#4597=EDGE_CURVE ( 'NONE', #10621, #505, #4675, .T. ) ;
#4598=PRODUCT_DEFINITION_FORMATION_WITH_SPECIFIED_SOURCE ( 'ANY', '', #6207, .NOT_KNOWN. ) ;
#4601=EDGE_LOOP ( 'NONE', ( #2614, #8320, #15118, #1286, #11380, #11831, #2461, #5985 ) ) ;
#4611=FACE_OUTER_BOUND ( 'NONE', #11896, .T. ) ;
#4624=LINE ( 'NONE', #11741, #5484 ) ;
#4626=DIRECTION ( 'NONE',  ( 1.000000000000000000, 0.000000000000000000, 0.000000000000000000 ) ) ;
#4630=ADVANCED_FACE ( 'NONE', ( #3748 ), #15056, .F. ) ;
#4636=EDGE_CURVE ( 'NONE', #4073, #2148, #6640, .T. ) ;
#4641=ORIENTED_EDGE ( 'NONE', *, *, #16668, .F. ) ;
#4643=B_SPLINE_CURVE_WITH_KNOTS ( 'NONE', 3,
 ( #18150, #5319, #1127, #6825, #5876, #10101, #2987, #8610, #266, #18442 ),
 .UNSPECIFIED., .F., .F.,
 ( 4, 2, 2, 2, 4 ),
 ( 0.0003974689443029659507, 0.008237140244579449141, 0.01019705806964857006, 0.01215697589471769098, 0.01607681154485594496 ),
 .UNSPECIFIED. ) ;
#4647=CARTESIAN_POINT ( 'NONE',  ( -66.13756785686383921, 112.1658165091852908, -26.33995503696884910 ) ) ;
#4668=CARTESIAN_POINT ( 'NONE',  ( -123.4618227840623632, -151.5628872026273086, -18.23991632971910803 ) ) ;
#4670=CYLINDRICAL_SURFACE ( 'NONE', #17317, 20.99999999999999645 ) ;
#4675=LINE ( 'NONE', #6076, #15539 ) ;
#4677=ADVANCED_FACE ( 'NONE', ( #17952 ), #10955, .F. ) ;
#4687=ORIENTED_EDGE ( 'NONE', *, *, #11548, .T. ) ;
#4693=CARTESIAN_POINT ( 'NONE',  ( -123.4618227840623632, -111.0842361345572158, 57.00000000000000000 ) ) ;
#4702=DIRECTION ( 'NONE',  ( -1.000000000000000000, -0.000000000000000000, -0.000000000000000000 ) ) ;
#4713=CARTESIAN_POINT ( 'NONE',  ( -100.4870060002411805, -151.5628872026273086, -57.00000000000000000 ) ) ;
#4714=ORIENTED_EDGE ( 'NONE', *, *, #8572, .F. ) ;
#4719=ORIENTED_EDGE ( 'NONE', *, *, #7223, .T. ) ;
#4726=CIRCLE ( 'NONE', #1459, 20.99999999999998934 ) ;
#4734=EDGE_LOOP ( 'NONE', ( #16114, #13054, #1104, #1885 ) ) ;
#4742=VERTEX_POINT ( 'NONE', #17859 ) ;
#4749=FACE_OUTER_BOUND ( 'NONE', #17039, .T. ) ;
#4751=CARTESIAN_POINT ( 'NONE',  ( -67.59262256747315689, 0.000000000000000000, 0.000000000000000000 ) ) ;
#4754=CARTESIAN_POINT ( 'NONE',  ( -46.00691148729628566, 49.61991837646342418, -27.56955468854675928 ) ) ;
#4755=PLANE ( 'NONE',  #13247 ) ;
#4761=ORIENTED_EDGE ( 'NONE', *, *, #8356, .F. ) ;
#4764=VECTOR ( 'NONE', #9735, 1000.000000000000000 ) ;
#4767=DIRECTION ( 'NONE',  ( 0.000000000000000000, 0.000000000000000000, -1.000000000000000000 ) ) ;
#4772=ORIENTED_EDGE ( 'NONE', *, *, #3097, .T. ) ;
#4778=CARTESIAN_POINT ( 'NONE',  ( -67.59262256747315689, 50.58224449241410525, -15.00000000000000711 ) ) ;
#4787=AXIS2_PLACEMENT_3D ( 'NONE', #9615, #15509, #5590 ) ;
#4812=VECTOR ( 'NONE', #16001, 1000.000000000000000 ) ;
#4813=EDGE_LOOP ( 'NONE', ( #13052, #9623, #3419, #5022 ) ) ;
#4845=CIRCLE ( 'NONE', #3066, 20.99999999999999645 ) ;
#4850=CIRCLE ( 'NONE', #15644, 81.86696747278378439 ) ;
#4855=EDGE_CURVE ( 'NONE', #1895, #12660, #8701, .T. ) ;
#4857=CARTESIAN_POINT ( 'NONE',  ( -76.13473419340549242, 61.88023627570096608, -26.63205224474248922 ) ) ;
#4866=AXIS2_PLACEMENT_3D ( 'NONE', #2068, #9276, #16369 ) ;
#4884=LINE ( 'NONE', #8922, #16698 ) ;
#4886=AXIS2_PLACEMENT_3D ( 'NONE', #9230, #16613, #17917 ) ;
#4915=VECTOR ( 'NONE', #9737, 1000.000000000000000 ) ;
#4917=AXIS2_PLACEMENT_3D ( 'NONE', #1218, #3743, #13846 ) ;
#4921=CARTESIAN_POINT ( 'NONE',  ( -102.4618227840623774, -151.5628872026273086, 36.00000000000000711 ) ) ;
#4926=EDGE_CURVE ( 'NONE', #7603, #11788, #11688, .T. ) ;
#4934=CARTESIAN_POINT ( 'NONE',  ( -100.4870060002411805, -151.5628872026273086, -18.23991632971910803 ) ) ;
#4936=EDGE_CURVE ( 'NONE', #3955, #2953, #6887, .T. ) ;
#4942=EDGE_CURVE ( 'NONE', #9953, #3055, #14066, .T. ) ;
#4943=CARTESIAN_POINT ( 'NONE',  ( -27.71117476891160081, 84.22855780814606419, 25.00000000000000355 ) ) ;
#4945=EDGE_LOOP ( 'NONE', ( #12875, #2162, #18139, #1356, #306, #7134, #3160, #10501, #16789, #4641, #11834, #504, #8194, #429, #18310, #9046 ) ) ;
#4946=ORIENTED_EDGE ( 'NONE', *, *, #17172, .F. ) ;
#4950=ORIENTED_EDGE ( 'NONE', *, *, #1456, .T. ) ;
#4953=CARTESIAN_POINT ( 'NONE',  ( -73.87934070579318302, 108.3200415776840515, 23.04436415747560574 ) ) ;
#4958=CARTESIAN_POINT ( 'NONE',  ( -75.54870230859340552, 61.39300225715819437, -24.42246604956295286 ) ) ;
#4966=CARTESIAN_POINT ( 'NONE',  ( -40.00733709395555593, 54.39356007051860331, -24.23452569059776351 ) ) ;
#4969=DIRECTION ( 'NONE',  ( 0.000000000000000000, -1.000000000000000000, 0.000000000000000000 ) ) ;
#4975=ORIENTED_EDGE ( 'NONE', *, *, #9355, .F. ) ;
#4977=ORIENTED_EDGE ( 'NONE', *, *, #4926, .T. ) ;
#4983=DIRECTION ( 'NONE',  ( 0.000000000000000000, 0.000000000000000000, 1.000000000000000000 ) ) ;
#4985=ORIENTED_EDGE ( 'NONE', *, *, #485, .T. ) ;
#4988=ORIENTED_EDGE ( 'NONE', *, *, #16020, .T. ) ;
#4993=FACE_OUTER_BOUND ( 'NONE', #15668, .T. ) ;
#4996=CARTESIAN_POINT ( 'NONE',  ( 124.5381772159375942, -151.5628872026272802, 36.00000000000000711 ) ) ;
#5000=AXIS2_PLACEMENT_3D ( 'NONE', #11984, #9098, #16285 ) ;
#5001=CARTESIAN_POINT ( 'NONE',  ( 5.233202738124664855, -19.34983604512936495, 54.79921157549230770 ) ) ;
#5006=LINE ( 'NONE', #12045, #17126 ) ;
#5008=ORIENTED_EDGE ( 'NONE', *, *, #9621, .F. ) ;
#5010=EDGE_CURVE ( 'NONE', #13442, #17304, #13763, .T. ) ;
#5014=CARTESIAN_POINT ( 'NONE',  ( 15.23320273812466574, -111.0842361345572158, 57.00000000000000000 ) ) ;
#5022=ORIENTED_EDGE ( 'NONE', *, *, #15806, .F. ) ;
#5030=FACE_OUTER_BOUND ( 'NONE', #8067, .T. ) ;
#5031=CARTESIAN_POINT ( 'NONE',  ( -70.64145177051501889, 58.17045213671937631, 22.35917033480641791 ) ) ;
#5035=CARTESIAN_POINT ( 'NONE',  ( -57.08002265617300708, 84.22855780814606419, -35.00000000000000000 ) ) ;
#5039=EDGE_LOOP ( 'NONE', ( #11130, #4687, #15225, #3802, #10640, #1606, #18307, #12488 ) ) ;
#5040=CARTESIAN_POINT ( 'NONE',  ( -72.62084357432196668, 59.30745156523346395, -22.61749258835635246 ) ) ;
#5047=EDGE_CURVE ( 'NONE', #18453, #7572, #3815, .T. ) ;
#5053=CARTESIAN_POINT ( 'NONE',  ( -41.66054475863654716, 53.50644796006596948, -24.87164372060468764 ) ) ;
#5056=CARTESIAN_POINT ( 'NONE',  ( -123.4618227840623632, -151.5628872026273086, 18.23991632971911514 ) ) ;
#5070=AXIS2_PLACEMENT_3D ( 'NONE', #4301, #12542, #6734 ) ;
#5072=CARTESIAN_POINT ( 'NONE',  ( -67.59262256747319952, 110.5691553257988460, 26.35917033480641436 ) ) ;
#5079=ORIENTED_EDGE ( 'NONE', *, *, #2544, .T. ) ;
#5080=CARTESIAN_POINT ( 'NONE',  ( 5.233202738124664855, -111.0842361345572158, 57.00000000000000000 ) ) ;
#5089=CIRCLE ( 'NONE', #16453, 3.999999999999989786 ) ;
#5090=CARTESIAN_POINT ( 'NONE',  ( -83.12361985383351737, 84.22855780814606419, -47.49999999999999289 ) ) ;
#5099=ORIENTED_EDGE ( 'NONE', *, *, #10087, .F. ) ;
#5102=DIRECTION ( 'NONE',  ( -1.000000000000000000, 0.000000000000000000, 1.156482317317869999E-16 ) ) ;
#5110=ORIENTED_EDGE ( 'NONE', *, *, #18430, .F. ) ;
#5114=CARTESIAN_POINT ( 'NONE',  ( -127.5926225674731711, 57.88796029049329661, 30.35917033480640370 ) ) ;
#5128=CARTESIAN_POINT ( 'NONE',  ( -66.06069454268705954, 57.36660113903539582, 25.00000000000000355 ) ) ;
#5137=DIRECTION ( 'NONE',  ( -1.000000000000000000, -0.000000000000000000, -0.000000000000000000 ) ) ;
#5147=ADVANCED_FACE ( 'NONE', ( #14928 ), #2129, .F. ) ;
#5149=EDGE_CURVE ( 'NONE', #14649, #3187, #3021, .T. ) ;
#5172=EDGE_CURVE ( 'NONE', #13683, #10531, #2110, .T. ) ;
#5174=VECTOR ( 'NONE', #2328, 1000.000000000000000 ) ;
#5175=AXIS2_PLACEMENT_3D ( 'NONE', #8601, #2515, #9622 ) ;
#5183=CARTESIAN_POINT ( 'NONE',  ( -67.59262256747315689, 0.000000000000000000, 0.000000000000000000 ) ) ;
#5190=CARTESIAN_POINT ( 'NONE',  ( -76.09664428591263174, 106.6093187847199459, -26.96894390707464240 ) ) ;
#5196=AXIS2_PLACEMENT_3D ( 'NONE', #2710, #2619, #15797 ) ;
#5201=PLANE ( 'NONE',  #11394 ) ;
#5204=CYLINDRICAL_SURFACE ( 'NONE', #18362, 170.8515291679562154 ) ;
#5205=ORIENTED_EDGE ( 'NONE', *, *, #12596, .T. ) ;
#5215=AXIS2_PLACEMENT_3D ( 'NONE', #17065, #2580, #15573 ) ;
#5216=AXIS2_PLACEMENT_3D ( 'NONE', #7048, #14049, #12664 ) ;
#5226=AXIS2_PLACEMENT_3D ( 'NONE', #9533, #15050, #3922 ) ;
#5228=LINE ( 'NONE', #18342, #3436 ) ;
#5231=LINE ( 'NONE', #10950, #13455 ) ;
#5233=CYLINDRICAL_SURFACE ( 'NONE', #13597, 26.04359719766049253 ) ;
#5234=DIRECTION ( 'NONE',  ( 0.000000000000000000, 0.000000000000000000, -1.000000000000000000 ) ) ;
#5236=EDGE_CURVE ( 'NONE', #11287, #9128, #17425, .T. ) ;
#5244=ORIENTED_EDGE ( 'NONE', *, *, #6145, .T. ) ;
#5255=ORIENTED_EDGE ( 'NONE', *, *, #16936, .F. ) ;
#5257=CARTESIAN_POINT ( 'NONE',  ( -92.59262256747319952, 57.88796029049329661, 22.35917033480642502 ) ) ;
#5266=FACE_OUTER_BOUND ( 'NONE', #3404, .T. ) ;
#5271=EDGE_CURVE ( 'NONE', #8070, #1253, #5588, .T. ) ;
#5288=EDGE_LOOP ( 'NONE', ( #7629, #16532, #9236, #6598 ) ) ;
#5294=DIRECTION ( 'NONE',  ( -0.000000000000000000, -0.000000000000000000, 1.000000000000000000 ) ) ;
#5299=LINE ( 'NONE', #10927, #10554 ) ;
#5306=DIRECTION ( 'NONE',  ( -1.000000000000000000, -1.119176436114069332E-16, 0.000000000000000000 ) ) ;
#5310=DIRECTION ( 'NONE',  ( 0.000000000000000000, 0.000000000000000000, -1.000000000000000000 ) ) ;
#5319=CARTESIAN_POINT ( 'NONE',  ( -47.50120849787443689, 51.11741075767032783, 26.54703875325328966 ) ) ;
#5321=ORIENTED_EDGE ( 'NONE', *, *, #9877, .F. ) ;
#5350=ORIENTED_EDGE ( 'NONE', *, *, #10087, .T. ) ;
#5356=CARTESIAN_POINT ( 'NONE',  ( 5.090901028739964751, 20.32480939964089117, -43.45823631389497876 ) ) ;
#5359=DIRECTION ( 'NONE',  ( 1.000000000000000000, 0.000000000000000000, 0.000000000000000000 ) ) ;
#5370=PLANE ( 'NONE',  #8821 ) ;
#5379=DIRECTION ( 'NONE',  ( -0.000000000000000000, 1.000000000000000000, -0.000000000000000000 ) ) ;
#5380=CARTESIAN_POINT ( 'NONE',  ( -64.09025127992791226, 117.8748711238780373, -35.00000000000000000 ) ) ;
#5381=ORIENTED_EDGE ( 'NONE', *, *, #13065, .F. ) ;
#5389=ORIENTED_EDGE ( 'NONE', *, *, #1507, .F. ) ;
#5390=EDGE_CURVE ( 'NONE', #18482, #1708, #3389, .T. ) ;
#5393=( NAMED_UNIT ( * ) PLANE_ANGLE_UNIT ( ) SI_UNIT ( $, .RADIAN. ) );
#5401=AXIS2_PLACEMENT_3D ( 'NONE', #2225, #3618, #7938 ) ;
#5406=ORIENTED_EDGE ( 'NONE', *, *, #17178, .F. ) ;
#5407=EDGE_LOOP ( 'NONE', ( #14144, #12511, #2777, #2302, #7802, #9527, #13802, #17295, #9895, #8177, #14323, #7641 ) ) ;
#5410=DIRECTION ( 'NONE',  ( -0.000000000000000000, -0.000000000000000000, -1.000000000000000000 ) ) ;
#5415=AXIS2_PLACEMENT_3D ( 'NONE', #2476, #9780, #3871 ) ;
#5426=VERTEX_POINT ( 'NONE', #17702 ) ;
#5431=CARTESIAN_POINT ( 'NONE',  ( -44.49764538373973721, 84.22855780814606419, 37.50000000000000000 ) ) ;
#5434=DIRECTION ( 'NONE',  ( -0.000000000000000000, -0.000000000000000000, -1.000000000000000000 ) ) ;
#5438=EDGE_LOOP ( 'NONE', ( #17008, #17427, #15969, #10124 ) ) ;
#5440=DIRECTION ( 'NONE',  ( 0.000000000000000000, -4.000800291689476871E-17, -1.000000000000000000 ) ) ;
#5441=DIRECTION ( 'NONE',  ( 0.000000000000000000, 0.000000000000000000, -1.000000000000000000 ) ) ;
#5454=DIRECTION ( 'NONE',  ( -0.000000000000000000, -0.000000000000000000, 1.000000000000000000 ) ) ;
#5460=CARTESIAN_POINT ( 'NONE',  ( 8.584122944725191218, 13.03299671059484233, -46.30665401617704902 ) ) ;
#5461=DIRECTION ( 'NONE',  ( -0.000000000000000000, 1.000000000000000000, -0.000000000000000000 ) ) ;
#5463=VECTOR ( 'NONE', #3069, 1000.000000000000000 ) ;
#5465=CARTESIAN_POINT ( 'NONE',  ( -69.25984391241293281, 110.9679338156112323, 22.35917033480641791 ) ) ;
#5472=CIRCLE ( 'NONE', #3696, 20.99999999999998934 ) ;
#5484=VECTOR ( 'NONE', #15947, 1000.000000000000000 ) ;
#5492=CARTESIAN_POINT ( 'NONE',  ( -75.22571693091748557, 107.3221758769030458, 24.00774849279516232 ) ) ;
#5496=EDGE_CURVE ( 'NONE', #18453, #2768, #8318, .T. ) ;
#5503=CIRCLE ( 'NONE', #5196, 3.999999999999989786 ) ;
#5505=ORIENTED_EDGE ( 'NONE', *, *, #18382, .F. ) ;
#5510=FACE_OUTER_BOUND ( 'NONE', #11950, .T. ) ;
#5518=CARTESIAN_POINT ( 'NONE',  ( -66.32832664217301044, 109.6035164793382393, -28.00000000000000355 ) ) ;
#5522=CIRCLE ( 'NONE', #1932, 26.04359719766049608 ) ;
#5544=ORIENTED_EDGE ( 'NONE', *, *, #17275, .T. ) ;
#5557=ORIENTED_EDGE ( 'NONE', *, *, #12007, .T. ) ;
#5558=CARTESIAN_POINT ( 'NONE',  ( -23.71312654895687189, 50.37139919635580299, -27.05770456752418696 ) ) ;
#5562=CARTESIAN_POINT ( 'NONE',  ( -70.06856178257680767, 110.5691553257988460, 22.35917033480641791 ) ) ;
#5565=CARTESIAN_POINT ( 'NONE',  ( -70.47187574892673467, 110.3702813545971679, -22.35917033480642147 ) ) ;
#5571=DIRECTION ( 'NONE',  ( -0.9475106458593564041, -0.3197242186372270534, 0.000000000000000000 ) ) ;
#5573=CARTESIAN_POINT ( 'NONE',  ( -67.59262256747317110, 56.80567558672318995, 22.50837044127973030 ) ) ;
#5588=LINE ( 'NONE', #14021, #3520 ) ;
#5589=EDGE_CURVE ( 'NONE', #3055, #3490, #16959, .T. ) ;
#5590=DIRECTION ( 'NONE',  ( 1.000000000000000000, 0.000000000000000000, 0.000000000000000000 ) ) ;
#5592=ORIENTED_EDGE ( 'NONE', *, *, #12204, .T. ) ;
#5594=FACE_OUTER_BOUND ( 'NONE', #9691, .T. ) ;
#5602=CARTESIAN_POINT ( 'NONE',  ( 15.23320273812466041, -19.34983604512934363, 3.000000000000000000 ) ) ;
#5607=ADVANCED_FACE ( 'NONE', ( #5266 ), #14341, .F. ) ;
#5610=EDGE_CURVE ( 'NONE', #17762, #5426, #7412, .T. ) ;
#5633=CARTESIAN_POINT ( 'NONE',  ( 9.543663295069050534, 56.41207303426870112, 7.000000000000010658 ) ) ;
#5643=DIRECTION ( 'NONE',  ( 4.675871521838984962E-16, -1.000000000000000000, 0.000000000000000000 ) ) ;
#5645=ORIENTED_EDGE ( 'NONE', *, *, #1041, .T. ) ;
#5653=ORIENTED_EDGE ( 'NONE', *, *, #16946, .F. ) ;
#5659=VECTOR ( 'NONE', #994, 1000.000000000000000 ) ;
#5660=VERTEX_POINT ( 'NONE', #12954 ) ;
#5682=ORIENTED_EDGE ( 'NONE', *, *, #16936, .T. ) ;
#5686=CARTESIAN_POINT ( 'NONE',  ( -67.59262256747317110, 57.88796029049329661, 30.35917033480639660 ) ) ;
#5690=CARTESIAN_POINT ( 'NONE',  ( -66.75310480962880888, 108.5438542518999725, -28.00000000000000711 ) ) ;
#5697=DIRECTION ( 'NONE',  ( -0.000000000000000000, 1.000000000000000000, -0.000000000000000000 ) ) ;
#5698=EDGE_LOOP ( 'NONE', ( #14722, #5645, #3928, #16433 ) ) ;
#5707=CONICAL_SURFACE ( 'NONE', #45, 3.999999999999989786, 1.029744258676652091 ) ;
#5708=CARTESIAN_POINT ( 'NONE',  ( 95.45835937779683888, -32.62665103886254059, 7.000000000000010658 ) ) ;
#5715=ORIENTED_EDGE ( 'NONE', *, *, #3675, .T. ) ;
#5721=VERTEX_POINT ( 'NONE', #17578 ) ;
#5725=EDGE_CURVE ( 'NONE', #2362, #12457, #3470, .T. ) ;
#5740=ADVANCED_FACE ( 'NONE', ( #16179 ), #10123, .F. ) ;
#5769=CARTESIAN_POINT ( 'NONE',  ( -64.09025127992789805, 84.22855780814606419, 28.00000000000000355 ) ) ;
#5770=ORIENTED_EDGE ( 'NONE', *, *, #1041, .F. ) ;
#5773=DIRECTION ( 'NONE',  ( 1.000000000000000000, 0.000000000000000000, 0.000000000000000000 ) ) ;
#5781=CARTESIAN_POINT ( 'NONE',  ( 0.000000000000000000, 0.000000000000000000, 0.000000000000000000 ) ) ;
#5786=CARTESIAN_POINT ( 'NONE',  ( -68.12361985383350316, 84.22855780814606419, 37.50000000000000000 ) ) ;
#5801=B_SPLINE_CURVE_WITH_KNOTS ( 'NONE', 3,
 ( #11880, #4754, #9086, #1974, #11307, #1390, #16807, #8504, #16997, #8303, #8211, #14017, #14113, #12335, #15606, #7004, #11219, #4100, #9712, #18028, #13823, #18420, #12527, #9804, #14211, #2504, #13928, #1113 ),
 .UNSPECIFIED., .F., .F.,
 ( 4, 2, 2, 2, 2, 2, 2, 2, 2, 2, 2, 2, 2, 4 ),
 ( 0.000000000000000000, 0.01246990002149389425, 0.01870485003224084050, 0.02182232503761430756, 0.02493980004298777114, 0.03740970006448163937, 0.04364465007522858736, 0.04676212508060205442, 0.04987960008597552147, 0.06234950010746938276, 0.07481940012896323711, 0.08105435013971017122, 0.08728930015045711921, 0.09975920017195097356 ),
 .UNSPECIFIED. ) ;
#5803=CARTESIAN_POINT ( 'NONE',  ( -70.71978124295696944, -141.5628872026273086, 18.23991632971911514 ) ) ;
#5804=DIRECTION ( 'NONE',  ( -0.000000000000000000, -0.000000000000000000, -1.000000000000000000 ) ) ;
#5814=FACE_OUTER_BOUND ( 'NONE', #6725, .T. ) ;
#5830=EDGE_CURVE ( 'NONE', #4, #17405, #7765, .T. ) ;
#5843=EDGE_CURVE ( 'NONE', #2177, #7603, #4726, .T. ) ;
#5853=ORIENTED_EDGE ( 'NONE', *, *, #4855, .T. ) ;
#5861=DIRECTION ( 'NONE',  ( -0.000000000000000000, 0.000000000000000000, 1.000000000000000000 ) ) ;
#5864=CARTESIAN_POINT ( 'NONE',  ( -57.08002265617300708, 84.22855780814606419, -47.50000000000000000 ) ) ;
#5869=CARTESIAN_POINT ( 'NONE',  ( -64.09025127992788384, 59.14618053571278722, 28.00000000000000355 ) ) ;
#5870=( NAMED_UNIT ( * ) SI_UNIT ( $, .STERADIAN. ) SOLID_ANGLE_UNIT ( ) );
#5876=CARTESIAN_POINT ( 'NONE',  ( -41.64957301763954689, 53.51189571422416691, 24.86776167054292586 ) ) ;
#5877=CYLINDRICAL_SURFACE ( 'NONE', #1850, 3.999999999999996447 ) ;
#5885=ORIENTED_EDGE ( 'NONE', *, *, #11215, .T. ) ;
#5889=LINE ( 'NONE', #7312, #10721 ) ;
#5897=ORIENTED_EDGE ( 'NONE', *, *, #1163, .F. ) ;
#5901=ORIENTED_EDGE ( 'NONE', *, *, #13624, .T. ) ;
#5906=EDGE_LOOP ( 'NONE', ( #13535, #18494, #12945, #13795 ) ) ;
#5911=DIRECTION ( 'NONE',  ( 1.000000000000000000, 0.000000000000000000, 0.000000000000000000 ) ) ;
#5916=ORIENTED_EDGE ( 'NONE', *, *, #9268, .F. ) ;
#5920=ORIENTED_EDGE ( 'NONE', *, *, #14208, .T. ) ;
#5928=LINE ( 'NONE', #14371, #1817 ) ;
#5931=EDGE_LOOP ( 'NONE', ( #8368, #7347, #9008, #270, #13047, #12711 ) ) ;
#5935=CARTESIAN_POINT ( 'NONE',  ( -75.86129610575210336, 61.64996188551982925, 25.00000000000000355 ) ) ;
#5940=ADVANCED_FACE ( 'NONE', ( #847 ), #13759, .F. ) ;
#5952=CARTESIAN_POINT ( 'NONE',  ( -66.00585202009862940, 110.5691553257988460, 25.00000000000000355 ) ) ;
#5954=LINE ( 'NONE', #12916, #12595 ) ;
#5958=CARTESIAN_POINT ( 'NONE',  ( -127.5926225674731995, 110.5691553257988460, 26.35917033480641436 ) ) ;
#5965=VECTOR ( 'NONE', #18034, 1000.000000000000000 ) ;
#5971=VECTOR ( 'NONE', #2508, 1000.000000000000000 ) ;
#5974=DIRECTION ( 'NONE',  ( -0.000000000000000000, -0.000000000000000000, -1.000000000000000000 ) ) ;
#5985=ORIENTED_EDGE ( 'NONE', *, *, #7203, .T. ) ;
#5991=CARTESIAN_POINT ( 'NONE',  ( -66.40868851600845346, 56.38066346224191960, 25.00000000000000355 ) ) ;
#5995=AXIS2_PLACEMENT_3D ( 'NONE', #2861, #4424, #13056 ) ;
#5999=CARTESIAN_POINT ( 'NONE',  ( -123.4618227840623632, -151.5628872026273086, 36.00000000000001421 ) ) ;
#6000=CARTESIAN_POINT ( 'NONE',  ( 103.5381772159376084, -111.0842361345572158, -36.00000000000000000 ) ) ;
#6003=ORIENTED_EDGE ( 'NONE', *, *, #4260, .T. ) ;
#6012=CARTESIAN_POINT ( 'NONE',  ( -66.63376473465912397, -19.34983604512935429, 57.00000000000000000 ) ) ;
#6025=AXIS2_PLACEMENT_3D ( 'NONE', #12627, #18325, #5306 ) ;
#6037=DIRECTION ( 'NONE',  ( 0.000000000000000000, 0.000000000000000000, 1.000000000000000000 ) ) ;
#6044=CYLINDRICAL_SURFACE ( 'NONE', #15092, 71.86696747278378439 ) ;
#6049=CARTESIAN_POINT ( 'NONE',  ( 124.5381772159375942, -111.0842361345572158, -36.00000000000000000 ) ) ;
#6057=AXIS2_PLACEMENT_3D ( 'NONE', #11996, #12100, #13682 ) ;
#6063=ORIENTED_EDGE ( 'NONE', *, *, #15594, .T. ) ;
#6065=CARTESIAN_POINT ( 'NONE',  ( 5.233202738124664855, -19.34983604512936495, -54.79921157549230770 ) ) ;
#6069=DIRECTION ( 'NONE',  ( -1.000000000000000000, 0.000000000000000000, 0.000000000000000000 ) ) ;
#6073=ORIENTED_EDGE ( 'NONE', *, *, #1762, .T. ) ;
#6076=CARTESIAN_POINT ( 'NONE',  ( -123.4618227840623632, -111.0842361345572158, 57.00000000000000000 ) ) ;
#6083=VERTEX_POINT ( 'NONE', #17025 ) ;
#6090=CIRCLE ( 'NONE', #18376, 26.04359719766049608 ) ;
#6096=EDGE_LOOP ( 'NONE', ( #11888, #16382 ) ) ;
#6097=VECTOR ( 'NONE', #3352, 1000.000000000000000 ) ;
#6099=ORIENTED_EDGE ( 'NONE', *, *, #14208, .F. ) ;
#6104=VECTOR ( 'NONE', #8694, 1000.000000000000000 ) ;
#6107=FACE_OUTER_BOUND ( 'NONE', #7738, .T. ) ;
#6115=CARTESIAN_POINT ( 'NONE',  ( -57.08002265617300708, 84.22855780814606419, -28.00000000000000355 ) ) ;
#6132=DIRECTION ( 'NONE',  ( -1.000000000000000000, 0.000000000000000000, 0.000000000000000000 ) ) ;
#6134=CARTESIAN_POINT ( 'NONE',  ( -127.5926225674731995, 106.8071537307722991, 25.00000000000000355 ) ) ;
#6136=ORIENTED_EDGE ( 'NONE', *, *, #10317, .T. ) ;
#6137=DIRECTION ( 'NONE',  ( 1.000000000000000000, 0.000000000000000000, 0.000000000000000000 ) ) ;
#6138=VERTEX_POINT ( 'NONE', #1502 ) ;
#6145=EDGE_CURVE ( 'NONE', #8271, #3955, #14645, .T. ) ;
#6152=EDGE_CURVE ( 'NONE', #17871, #5721, #13363, .T. ) ;
#6176=CARTESIAN_POINT ( 'NONE',  ( -67.59262256747319952, 106.8071537307723133, 25.00000000000000355 ) ) ;
#6177=LINE ( 'NONE', #7786, #12300 ) ;
#6199=CARTESIAN_POINT ( 'NONE',  ( -57.08002265617300708, 84.22855780814606419, 37.50000000000000000 ) ) ;
#6202=CARTESIAN_POINT ( 'NONE',  ( -67.59262256747319952, 111.6514400295689171, -22.50837044127971254 ) ) ;
#6204=DIRECTION ( 'NONE',  ( 0.000000000000000000, -0.000000000000000000, 1.000000000000000000 ) ) ;
#6207=PRODUCT ( 'C-Frame Forged Steel Casing', 'C-Frame Forged Steel Casing', '', ( #6575 ) ) ;
#6213=EDGE_LOOP ( 'NONE', ( #15633, #15761, #17600, #16394, #5901, #9185, #6243, #14935 ) ) ;
#6222=DIRECTION ( 'NONE',  ( -0.000000000000000000, -0.000000000000000000, -1.000000000000000000 ) ) ;
#6228=DIRECTION ( 'NONE',  ( -0.000000000000000000, 1.200240087506842815E-16, 1.000000000000000000 ) ) ;
#6229=ORIENTED_EDGE ( 'NONE', *, *, #8997, .F. ) ;
#6230=CARTESIAN_POINT ( 'NONE',  ( -66.00585202009801833, 57.88796029049324687, 25.00000000000000355 ) ) ;
#6232=AXIS2_PLACEMENT_3D ( 'NONE', #13998, #11288, #11193 ) ;
#6242=DIRECTION ( 'NONE',  ( 1.000000000000000000, 0.000000000000000000, 0.000000000000000000 ) ) ;
#6243=ORIENTED_EDGE ( 'NONE', *, *, #17224, .F. ) ;
#6246=ADVANCED_FACE ( 'NONE', ( #1021 ), #11129, .F. ) ;
#6247=DIRECTION ( 'NONE',  ( -1.000000000000000000, 0.000000000000000000, -0.000000000000000000 ) ) ;
#6251=FACE_OUTER_BOUND ( 'NONE', #14691, .T. ) ;
#6252=CARTESIAN_POINT ( 'NONE',  ( -67.59262256747317110, 56.80567558672318995, 22.50837044127973030 ) ) ;
#6253=ORIENTED_EDGE ( 'NONE', *, *, #14755, .T. ) ;
#6262=DIRECTION ( 'NONE',  ( -1.000000000000000000, 0.000000000000000000, -0.000000000000000000 ) ) ;
#6275=EDGE_LOOP ( 'NONE', ( #3578, #2316, #241, #1008, #15196, #503 ) ) ;
#6285=VERTEX_POINT ( 'NONE', #11503 ) ;
#6305=AXIS2_PLACEMENT_3D ( 'NONE', #14681, #6535, #3542 ) ;
#6316=ORIENTED_EDGE ( 'NONE', *, *, #4260, .F. ) ;
#6319=AXIS2_PLACEMENT_3D ( 'NONE', #11247, #15142, #15237 ) ;
#6320=FACE_OUTER_BOUND ( 'NONE', #4945, .T. ) ;
#6322=DIRECTION ( 'NONE',  ( -1.000000000000000000, 0.000000000000000000, 0.000000000000000000 ) ) ;
#6323=CARTESIAN_POINT ( 'NONE',  ( -17.00234300178814451, 45.78782387526246112, 30.07809993627739331 ) ) ;
#6325=CARTESIAN_POINT ( 'NONE',  ( -57.08002265617300708, 84.22855780814606419, -47.49999999999999289 ) ) ;
#6326=CARTESIAN_POINT ( 'NONE',  ( -57.08002265617300708, 84.22855780814606419, 35.00000000000000000 ) ) ;
#6334=VECTOR ( 'NONE', #2669, 1000.000000000000000 ) ;
#6335=FACE_OUTER_BOUND ( 'NONE', #5039, .T. ) ;
#6343=PLANE ( 'NONE',  #12934 ) ;
#6345=CARTESIAN_POINT ( 'NONE',  ( 0.000000000000000000, 0.000000000000000000, 57.00000000000000000 ) ) ;
#6353=ORIENTED_EDGE ( 'NONE', *, *, #934, .T. ) ;
#6363=EDGE_LOOP ( 'NONE', ( #986, #16904, #13409, #806, #4111, #1458 ) ) ;
#6364=LINE ( 'NONE', #5056, #17308 ) ;
#6369=FACE_OUTER_BOUND ( 'NONE', #7235, .T. ) ;
#6374=VERTEX_POINT ( 'NONE', #14299 ) ;
#6386=DIRECTION ( 'NONE',  ( 0.000000000000000000, 0.000000000000000000, 1.000000000000000000 ) ) ;
#6390=CARTESIAN_POINT ( 'NONE',  ( -83.12361985383351737, 84.22855780814606419, -35.00000000000000711 ) ) ;
#6393=DIRECTION ( 'NONE',  ( -0.000000000000000000, -1.000000000000000000, -0.000000000000000000 ) ) ;
#6397=CYLINDRICAL_SURFACE ( 'NONE', #9927, 26.04359719766049253 ) ;
#6401=VECTOR ( 'NONE', #2256, 1000.000000000000000 ) ;
#6402=B_SPLINE_CURVE_WITH_KNOTS ( 'NONE', 3,
 ( #14695, #7598, #491, #4966, #16371, #5053, #10771, #13218, #16465, #397 ),
 .UNSPECIFIED., .F., .F.,
 ( 4, 2, 2, 2, 4 ),
 ( 0.006898123196567208619, 0.01082895749156352269, 0.01279437463906168276, 0.01475979178655984284, 0.02262146037655243455 ),
 .UNSPECIFIED. ) ;
#6403=LINE ( 'NONE', #713, #10015 ) ;
#6409=VECTOR ( 'NONE', #15437, 1000.000000000000000 ) ;
#6412=EDGE_CURVE ( 'NONE', #2362, #11975, #15867, .T. ) ;
#6416=EDGE_LOOP ( 'NONE', ( #11296, #3575, #10565, #14583 ) ) ;
#6418=CARTESIAN_POINT ( 'NONE',  ( 4.873448657480574653, -11.10503745953439569, 53.31400367155413278 ) ) ;
#6431=DIRECTION ( 'NONE',  ( -1.000000000000000000, -0.000000000000000000, -0.000000000000000000 ) ) ;
#6440=ORIENTED_EDGE ( 'NONE', *, *, #18454, .T. ) ;
#6442=LINE ( 'NONE', #12162, #6097 ) ;
#6449=CARTESIAN_POINT ( 'NONE',  ( -73.36356571042369978, 59.78633783786654021, -22.83555841014880272 ) ) ;
#6456=CARTESIAN_POINT ( 'NONE',  ( 124.5381772159375942, -46.83756720124470263, 115.7605492041889619 ) ) ;
#6459=EDGE_CURVE ( 'NONE', #1208, #8420, #4077, .T. ) ;
#6480=DIRECTION ( 'NONE',  ( 0.000000000000000000, 1.000000000000000000, 0.000000000000000000 ) ) ;
#6481=ORIENTED_EDGE ( 'NONE', *, *, #11095, .F. ) ;
#6486=CARTESIAN_POINT ( 'NONE',  ( -67.25621515281476093, 107.4062629095552808, 25.00000000000000355 ) ) ;
#6493=ADVANCED_FACE ( 'NONE', ( #15285 ), #16774, .F. ) ;
#6495=EDGE_CURVE ( 'NONE', #12009, #2102, #9779, .T. ) ;
#6499=VERTEX_POINT ( 'NONE', #11284 ) ;
#6510=DIRECTION ( 'NONE',  ( -0.000000000000000000, -0.000000000000000000, 1.000000000000000000 ) ) ;
#6514=EDGE_CURVE ( 'NONE', #12457, #10530, #1245, .T. ) ;
#6535=DIRECTION ( 'NONE',  ( 0.000000000000000000, 0.000000000000000000, 1.000000000000000000 ) ) ;
#6541=ORIENTED_EDGE ( 'NONE', *, *, #14261, .F. ) ;
#6542=CARTESIAN_POINT ( 'NONE',  ( -67.59262256747315689, 129.5689604715732912, -15.00000000000001066 ) ) ;
#6543=CARTESIAN_POINT ( 'NONE',  ( -194.4437806548868934, -151.5628872026273086, 18.23991632971911869 ) ) ;
#6546=ORIENTED_EDGE ( 'NONE', *, *, #17152, .F. ) ;
#6551=DIRECTION ( 'NONE',  ( -1.000000000000000000, 0.000000000000000000, 0.000000000000000000 ) ) ;
#6568=PRODUCT_DEFINITION ( 'UNKNOWN', '', #4598, #13581 ) ;
#6570=AXIS2_PLACEMENT_3D ( 'NONE', #6831, #2721, #2824 ) ;
#6575=PRODUCT_CONTEXT ( 'NONE', #13873, 'mechanical' ) ;
#6578=VECTOR ( 'NONE', #537, 1000.000000000000000 ) ;
#6582=DIRECTION ( 'NONE',  ( -0.000000000000000000, -0.000000000000000000, -1.000000000000000000 ) ) ;
#6586=CARTESIAN_POINT ( 'NONE',  ( -76.06755393367096474, 106.6341280094858490, -25.60850497571804496 ) ) ;
#6590=VECTOR ( 'NONE', #2367, 1000.000000000000000 ) ;
#6598=ORIENTED_EDGE ( 'NONE', *, *, #8272, .T. ) ;
#6605=VECTOR ( 'NONE', #17225, 1000.000000000000000 ) ;
#6610=LINE ( 'NONE', #15126, #7243 ) ;
#6613=VECTOR ( 'NONE', #15910, 1000.000000000000000 ) ;
#6618=FACE_OUTER_BOUND ( 'NONE', #14555, .T. ) ;
#6627=AXIS2_PLACEMENT_3D ( 'NONE', #2219, #12440, #6715 ) ;
#6628=CIRCLE ( 'NONE', #14127, 12.58237727243326987 ) ;
#6631=CARTESIAN_POINT ( 'NONE',  ( -66.20309715099607217, 56.86452048533069359, 24.99999999999999645 ) ) ;
#6640=LINE ( 'NONE', #1132, #1787 ) ;
#6642=ORIENTED_EDGE ( 'NONE', *, *, #17478, .T. ) ;
#6645=AXIS2_PLACEMENT_3D ( 'NONE', #2764, #17163, #2584 ) ;
#6646=DIRECTION ( 'NONE',  ( 1.000000000000000000, 0.000000000000000000, 0.000000000000000000 ) ) ;
#6654=VECTOR ( 'NONE', #11159, 1000.000000000000000 ) ;
#6655=FACE_OUTER_BOUND ( 'NONE', #11314, .T. ) ;
#6657=DIRECTION ( 'NONE',  ( -1.000000000000000000, -0.000000000000000000, -0.000000000000000000 ) ) ;
#6672=ORIENTED_EDGE ( 'NONE', *, *, #11265, .F. ) ;
#6683=FACE_OUTER_BOUND ( 'NONE', #1744, .T. ) ;
#6686=CYLINDRICAL_SURFACE ( 'NONE', #5415, 81.86696747278379860 ) ;
#6687=DIRECTION ( 'NONE',  ( -1.000000000000000000, 0.000000000000000000, 0.000000000000000000 ) ) ;
#6689=AXIS2_PLACEMENT_3D ( 'NONE', #14283, #15946, #4436 ) ;
#6695=VERTEX_POINT ( 'NONE', #13319 ) ;
#6699=PRODUCT_DEFINITION_SHAPE ( 'NONE', 'NONE',  #6568 ) ;
#6704=DIRECTION ( 'NONE',  ( -1.000000000000000000, 0.000000000000000000, 1.156482317317869999E-16 ) ) ;
#6709=ADVANCED_FACE ( 'NONE', ( #13496 ), #679, .T. ) ;
#6715=DIRECTION ( 'NONE',  ( 0.000000000000000000, 0.000000000000000000, 1.000000000000000000 ) ) ;
#6719=AXIS2_PLACEMENT_3D ( 'NONE', #11871, #3630, #11962 ) ;
#6723=CARTESIAN_POINT ( 'NONE',  ( -57.08002265617300708, 106.8109350805793270, 25.00000000000000355 ) ) ;
#6725=EDGE_LOOP ( 'NONE', ( #16733, #17473, #2172, #15925 ) ) ;
#6726=VERTEX_POINT ( 'NONE', #9196 ) ;
#6729=AXIS2_PLACEMENT_3D ( 'NONE', #2760, #14177, #1367 ) ;
#6734=DIRECTION ( 'NONE',  ( -1.000000000000000000, -1.119176436114069332E-16, 0.000000000000000000 ) ) ;
#6737=CARTESIAN_POINT ( 'NONE',  ( -92.59262256747319952, 50.58224449241410525, -35.00000000000000000 ) ) ;
#6748=VERTEX_POINT ( 'NONE', #6176 ) ;
#6749=VERTEX_POINT ( 'NONE', #13129 ) ;
#6750=EDGE_CURVE ( 'NONE', #1922, #4543, #5089, .T. ) ;
#6751=DIRECTION ( 'NONE',  ( -0.000000000000000000, -0.000000000000000000, -1.000000000000000000 ) ) ;
#6763=ORIENTED_EDGE ( 'NONE', *, *, #9851, .F. ) ;
#6764=CARTESIAN_POINT ( 'NONE',  ( -67.59262256747317110, 57.88796029049329661, -26.35917033480641436 ) ) ;
#6777=EDGE_LOOP ( 'NONE', ( #3979, #8991, #4544, #15238 ) ) ;
#6779=CARTESIAN_POINT ( 'NONE',  ( -18.64094200358713493, 47.00521434539033550, -29.29675916631614285 ) ) ;
#6780=EDGE_CURVE ( 'NONE', #1253, #535, #1897, .T. ) ;
#6783=DIRECTION ( 'NONE',  ( 0.9475106458593564041, 0.3197242186372270534, 0.000000000000000000 ) ) ;
#6790=DIRECTION ( 'NONE',  ( 1.000000000000000000, 0.000000000000000000, 0.000000000000000000 ) ) ;
#6800=CARTESIAN_POINT ( 'NONE',  ( -15.48721883272544275, 31.28870489046039438, 38.35419603998612814 ) ) ;
#6811=CARTESIAN_POINT ( 'NONE',  ( -127.5926225674732279, 117.8748711238780373, 15.00000000000004263 ) ) ;
#6813=ORIENTED_EDGE ( 'NONE', *, *, #5843, .F. ) ;
#6818=EDGE_LOOP ( 'NONE', ( #2036, #10513, #13781, #6063, #5897, #17819, #9337, #14846, #9289, #13240, #938, #16181, #1596, #231, #1392, #8251 ) ) ;
#6820=CARTESIAN_POINT ( 'NONE',  ( -74.58996131697591636, 60.64882399698279869, 23.45497070566349507 ) ) ;
#6824=CARTESIAN_POINT ( 'NONE',  ( -64.09025127992788384, 59.14618053571278722, 37.50000000000000000 ) ) ;
#6825=CARTESIAN_POINT ( 'NONE',  ( -42.21392442226139252, 53.23479276110153791, 25.06499217785701461 ) ) ;
#6826=DIRECTION ( 'NONE',  ( -1.000000000000000000, 0.000000000000000000, 0.000000000000000000 ) ) ;
#6828=CARTESIAN_POINT ( 'NONE',  ( -70.06856178257687873, 57.88796029049330372, -22.35917033480642502 ) ) ;
#6830=VERTEX_POINT ( 'NONE', #5257 ) ;
#6831=CARTESIAN_POINT ( 'NONE',  ( 124.5381772159375942, -46.83756720124470263, -115.7605492041889619 ) ) ;
#6840=LINE ( 'NONE', #8049, #6654 ) ;
#6841=EDGE_CURVE ( 'NONE', #3187, #9439, #777, .T. ) ;
#6847=LINE ( 'NONE', #963, #9611 ) ;
#6851=CARTESIAN_POINT ( 'NONE',  ( -123.4618227840623632, -111.0842361345572158, -35.99999999999997158 ) ) ;
#6860=CARTESIAN_POINT ( 'NONE',  ( -69.66239992860627694, 84.22855780814606419, 37.50000000000000000 ) ) ;
#6868=CARTESIAN_POINT ( 'NONE',  ( -21.99673296352410645, 49.28519306194654348, -27.79101546118255328 ) ) ;
#6876=CARTESIAN_POINT ( 'NONE',  ( -70.87062273247055089, 110.1621498490178226, -22.37384807337301496 ) ) ;
#6878=ORIENTED_EDGE ( 'NONE', *, *, #5236, .T. ) ;
#6879=EDGE_CURVE ( 'NONE', #565, #10632, #4261, .T. ) ;
#6882=CARTESIAN_POINT ( 'NONE',  ( -66.14871330646369074, 56.29489271423182828, -26.09800720142019159 ) ) ;
#6887=CIRCLE ( 'NONE', #9886, 29.36884788726140627 ) ;
#6899=CARTESIAN_POINT ( 'NONE',  ( -75.86129610575210336, 106.8071537307722991, 25.00000000000000355 ) ) ;
#6901=CARTESIAN_POINT ( 'NONE',  ( 5.099753278416039315, 20.30794007945024759, 43.46515485487502417 ) ) ;
#6931=DIRECTION ( 'NONE',  ( 1.119176436114069332E-16, -1.000000000000000000, -0.000000000000000000 ) ) ;
#6935=CIRCLE ( 'NONE', #18285, 29.36884788726140627 ) ;
#6942=CIRCLE ( 'NONE', #17377, 12.58237727243326987 ) ;
#6954=DIRECTION ( 'NONE',  ( -1.000000000000000000, -0.000000000000000000, -0.000000000000000000 ) ) ;
#6958=VERTEX_POINT ( 'NONE', #12566 ) ;
#6976=VERTEX_POINT ( 'NONE', #12185 ) ;
#6980=CIRCLE ( 'NONE', #17410, 172.7605492041889192 ) ;
#6987=DIRECTION ( 'NONE',  ( 0.000000000000000000, 0.000000000000000000, -1.000000000000000000 ) ) ;
#7004=CARTESIAN_POINT ( 'NONE',  ( -11.55310279070829260, 26.82330587308622682, -40.51155826455459419 ) ) ;
#7011=EDGE_CURVE ( 'NONE', #3213, #13490, #1430, .T. ) ;
#7026=CIRCLE ( 'NONE', #12997, 3.999999999999989786 ) ;
#7027=CARTESIAN_POINT ( 'NONE',  ( -67.37304936704279612, 107.3218817776568130, -27.99999999999999645 ) ) ;
#7029=DIRECTION ( 'NONE',  ( -0.5150380749100570421, 1.049727191138616600E-16, -0.8571673007021106683 ) ) ;
#7048=CARTESIAN_POINT ( 'NONE',  ( -70.71978124295696944, -141.5628872026273086, 5.204170427930421283E-15 ) ) ;
#7049=CARTESIAN_POINT ( 'NONE',  ( -64.09025127992788384, 50.58224449241410525, 35.00000000000000000 ) ) ;
#7050=PLANE ( 'NONE',  #870 ) ;
#7059=ORIENTED_EDGE ( 'NONE', *, *, #17385, .F. ) ;
#7069=CARTESIAN_POINT ( 'NONE',  ( -17.02762337565411244, 45.80709108728513712, -30.06585831480913740 ) ) ;
#7070=CARTESIAN_POINT ( 'NONE',  ( -70.85175816390371040, -141.5628872026273086, -18.23991632971912225 ) ) ;
#7077=ORIENTED_EDGE ( 'NONE', *, *, #485, .F. ) ;
#7079=CARTESIAN_POINT ( 'NONE',  ( -67.36171047226943642, 56.71715511495233386, -22.93244165942064683 ) ) ;
#7085=CARTESIAN_POINT ( 'NONE',  ( 9.543663295069050534, 56.41207303426870112, 7.000000000000010658 ) ) ;
#7088=CARTESIAN_POINT ( 'NONE',  ( -123.4618227840623632, -111.0842361345572158, 57.00000000000000000 ) ) ;
#7091=VERTEX_POINT ( 'NONE', #11442 ) ;
#7096=ORIENTED_EDGE ( 'NONE', *, *, #9621, .T. ) ;
#7102=ADVANCED_FACE ( 'NONE', ( #18465 ), #14253, .F. ) ;
#7107=CARTESIAN_POINT ( 'NONE',  ( -75.73737094285307592, 61.54687875405910091, 24.71467968727341713 ) ) ;
#7108=DIRECTION ( 'NONE',  ( 1.000000000000000000, 0.000000000000000000, 0.000000000000000000 ) ) ;
#7109=ORIENTED_EDGE ( 'NONE', *, *, #1163, .T. ) ;
#7112=CARTESIAN_POINT ( 'NONE',  ( 113.3630170098443273, -111.0842361345571874, 7.000000000000010658 ) ) ;
#7116=CARTESIAN_POINT ( 'NONE',  ( -57.08002265617300708, 84.22855780814606419, 37.50000000000000000 ) ) ;
#7119=EDGE_LOOP ( 'NONE', ( #16844, #7372 ) ) ;
#7134=ORIENTED_EDGE ( 'NONE', *, *, #5610, .T. ) ;
#7135=CARTESIAN_POINT ( 'NONE',  ( 276.3098885457529832, -32.62665103886256190, 7.000000000000010658 ) ) ;
#7150=CYLINDRICAL_SURFACE ( 'NONE', #5215, 20.99999999999999645 ) ;
#7155=VERTEX_POINT ( 'NONE', #17669 ) ;
#7156=CARTESIAN_POINT ( 'NONE',  ( -50.41499038512538533, 117.9449492212793302, 0.000000000000000000 ) ) ;
#7158=ORIENTED_EDGE ( 'NONE', *, *, #1456, .F. ) ;
#7168=DIRECTION ( 'NONE',  ( -1.000000000000000000, -0.000000000000000000, -0.000000000000000000 ) ) ;
#7171=CIRCLE ( 'NONE', #6232, 29.36884788726140627 ) ;
#7174=LINE ( 'NONE', #8943, #3597 ) ;
#7178=CARTESIAN_POINT ( 'NONE',  ( 10.09176930091618196, 9.223890154941049246, 47.65417223256151402 ) ) ;
#7180=CARTESIAN_POINT ( 'NONE',  ( -70.71978124295696944, -111.0842361345572158, 18.23991632971911869 ) ) ;
#7192=CARTESIAN_POINT ( 'NONE',  ( -66.42454906961714300, 112.0712930187555827, -27.77368723278591744 ) ) ;
#7197=PLANE ( 'NONE',  #14651 ) ;
#7203=EDGE_CURVE ( 'NONE', #16062, #8476, #1255, .T. ) ;
#7213=ADVANCED_FACE ( 'NONE', ( #1693 ), #1877, .F. ) ;
#7218=LINE ( 'NONE', #14329, #10851 ) ;
#7219=DIRECTION ( 'NONE',  ( -1.000000000000000000, -1.119176436114069332E-16, 0.000000000000000000 ) ) ;
#7223=EDGE_CURVE ( 'NONE', #1925, #18214, #5801, .T. ) ;
#7235=EDGE_LOOP ( 'NONE', ( #12002, #14232, #10575, #9047, #7096, #1172, #13328 ) ) ;
#7242=ORIENTED_EDGE ( 'NONE', *, *, #12576, .F. ) ;
#7243=VECTOR ( 'NONE', #6510, 1000.000000000000000 ) ;
#7260=VECTOR ( 'NONE', #11591, 1000.000000000000000 ) ;
#7282=VECTOR ( 'NONE', #3599, 1000.000000000000000 ) ;
#7286=LINE ( 'NONE', #10447, #7260 ) ;
#7287=CARTESIAN_POINT ( 'NONE',  ( -69.26154997389616597, 110.9670925573097833, -22.35917033480641791 ) ) ;
#7290=DIRECTION ( 'NONE',  ( -0.000000000000000000, -0.000000000000000000, 1.000000000000000000 ) ) ;
#7296=AXIS2_PLACEMENT_3D ( 'NONE', #1007, #13718, #7927 ) ;
#7304=VECTOR ( 'NONE', #5571, 1000.000000000000000 ) ;
#7310=DIRECTION ( 'NONE',  ( -4.675871521838984962E-16, 1.000000000000000000, 0.000000000000000000 ) ) ;
#7312=CARTESIAN_POINT ( 'NONE',  ( 95.45835937779682467, 4.463510241361116170E-14, 3.000000000000000000 ) ) ;
#7335=VECTOR ( 'NONE', #2331, 1000.000000000000000 ) ;
#7339=ORIENTED_EDGE ( 'NONE', *, *, #15713, .F. ) ;
#7342=CYLINDRICAL_SURFACE ( 'NONE', #13501, 3.999999999999989786 ) ;
#7347=ORIENTED_EDGE ( 'NONE', *, *, #9355, .T. ) ;
#7351=VERTEX_POINT ( 'NONE', #5935 ) ;
#7353=VECTOR ( 'NONE', #11518, 1000.000000000000000 ) ;
#7372=ORIENTED_EDGE ( 'NONE', *, *, #18318, .T. ) ;
#7380=DIRECTION ( 'NONE',  ( -0.000000000000000000, -0.000000000000000000, -1.000000000000000000 ) ) ;
#7389=ORIENTED_EDGE ( 'NONE', *, *, #10075, .F. ) ;
#7397=ORIENTED_EDGE ( 'NONE', *, *, #18075, .T. ) ;
#7412=CIRCLE ( 'NONE', #13386, 29.36884788726140627 ) ;
#7429=CARTESIAN_POINT ( 'NONE',  ( 0.000000000000000000, -111.0842361345572158, 3.000000000000000000 ) ) ;
#7434=CARTESIAN_POINT ( 'NONE',  ( -66.63376473465912397, -19.34983604512935429, 3.000000000000000000 ) ) ;
#7435=ORIENTED_EDGE ( 'NONE', *, *, #4242, .T. ) ;
#7442=ORIENTED_EDGE ( 'NONE', *, *, #11343, .F. ) ;
#7451=CIRCLE ( 'NONE', #882, 180.8515291679561585 ) ;
#7456=LINE ( 'NONE', #13176, #982 ) ;
#7459=ADVANCED_BREP_SHAPE_REPRESENTATION ( '', ( #12831, #16217 ), #2819 ) ;
#7461=LINE ( 'NONE', #13445, #13317 ) ;
#7463=DIRECTION ( 'NONE',  ( -1.000000000000000000, -0.000000000000000000, -0.000000000000000000 ) ) ;
#7468=CARTESIAN_POINT ( 'NONE',  ( -67.42374588395286139, 61.35112309735787761, 25.00000000000000355 ) ) ;
#7479=CARTESIAN_POINT ( 'NONE',  ( 15.23320273812466574, -111.0842361345572158, -57.00000000000000000 ) ) ;
#7500=FACE_OUTER_BOUND ( 'NONE', #14200, .T. ) ;
#7506=CARTESIAN_POINT ( 'NONE',  ( -92.59262256747321373, 110.5691553257988460, 26.35917033480641436 ) ) ;
#7507=DIRECTION ( 'NONE',  ( 0.000000000000000000, 1.000000000000000000, 0.000000000000000000 ) ) ;
#7516=ORIENTED_EDGE ( 'NONE', *, *, #6152, .F. ) ;
#7519=VERTEX_POINT ( 'NONE', #9129 ) ;
#7539=DIRECTION ( 'NONE',  ( 0.000000000000000000, 0.000000000000000000, 1.000000000000000000 ) ) ;
#7540=ORIENTED_EDGE ( 'NONE', *, *, #11329, .T. ) ;
#7543=ADVANCED_FACE ( 'NONE', ( #10432 ), #6397, .T. ) ;
#7545=EDGE_CURVE ( 'NONE', #3187, #3490, #12313, .T. ) ;
#7547=EDGE_CURVE ( 'NONE', #3088, #17119, #4243, .T. ) ;
#7554=ORIENTED_EDGE ( 'NONE', *, *, #6459, .T. ) ;
#7558=CYLINDRICAL_SURFACE ( 'NONE', #661, 12.58237727243326987 ) ;
#7572=VERTEX_POINT ( 'NONE', #14993 ) ;
#7573=ORIENTED_EDGE ( 'NONE', *, *, #16020, .F. ) ;
#7594=CIRCLE ( 'NONE', #17735, 170.8515291679562154 ) ;
#7597=LINE ( 'NONE', #8737, #12092 ) ;
#7598=CARTESIAN_POINT ( 'NONE',  ( -37.39761953508091352, 56.02837566180792805, -23.04006316738493609 ) ) ;
#7603=VERTEX_POINT ( 'NONE', #17992 ) ;
#7605=CARTESIAN_POINT ( 'NONE',  ( -92.59262256747321373, 117.8748711238780373, 35.00000000000000000 ) ) ;
#7607=CARTESIAN_POINT ( 'NONE',  ( -127.5926225674731711, 61.64996188551982925, 25.00000000000000355 ) ) ;
#7608=DIRECTION ( 'NONE',  ( 1.000000000000000000, 0.000000000000000000, 0.000000000000000000 ) ) ;
#7618=VERTEX_POINT ( 'NONE', #16208 ) ;
#7622=CIRCLE ( 'NONE', #452, 29.36884788726140627 ) ;
#7629=ORIENTED_EDGE ( 'NONE', *, *, #6459, .F. ) ;
#7633=CARTESIAN_POINT ( 'NONE',  ( -66.76796488546020214, 108.3135598836077094, 24.99999999999999645 ) ) ;
#7636=AXIS2_PLACEMENT_3D ( 'NONE', #1755, #7731, #17643 ) ;
#7637=DIRECTION ( 'NONE',  ( 1.000000000000000000, 2.062304371594500494E-16, -0.000000000000000000 ) ) ;
#7638=FACE_OUTER_BOUND ( 'NONE', #4229, .T. ) ;
#7641=ORIENTED_EDGE ( 'NONE', *, *, #12007, .F. ) ;
#7646=CARTESIAN_POINT ( 'NONE',  ( -67.59262256747315689, 50.58224449241410525, 35.00000000000000000 ) ) ;
#7651=CARTESIAN_POINT ( 'NONE',  ( 103.5381772159376084, -151.5628872026272802, 36.00000000000000711 ) ) ;
#7652=CARTESIAN_POINT ( 'NONE',  ( 95.45835937779683888, -32.62665103886256190, 7.000000000000010658 ) ) ;
#7655=EDGE_CURVE ( 'NONE', #11856, #18083, #6942, .T. ) ;
#7658=CARTESIAN_POINT ( 'NONE',  ( -66.46593056348568496, 59.53070700554641803, 24.99999999999999289 ) ) ;
#7659=DIRECTION ( 'NONE',  ( 0.000000000000000000, -1.000000000000000000, 1.181335735494911869E-16 ) ) ;
#7668=CARTESIAN_POINT ( 'NONE',  ( -74.36104963774657506, 107.9768795091070359, 23.30522882661994899 ) ) ;
#7673=ADVANCED_FACE ( 'NONE', ( #10793 ), #9638, .F. ) ;
#7675=CARTESIAN_POINT ( 'NONE',  ( -75.91242157673514157, 61.69241362573040988, -27.61362678897647172 ) ) ;
#7677=ORIENTED_EDGE ( 'NONE', *, *, #9852, .T. ) ;
#7694=PLANE ( 'NONE',  #6057 ) ;
#7695=CARTESIAN_POINT ( 'NONE',  ( -64.09025127992791226, 117.8748711238780373, 35.00000000000000000 ) ) ;
#7697=CARTESIAN_POINT ( 'NONE',  ( -123.4618227840623632, -151.5628872026273086, 18.23991632971911869 ) ) ;
#7698=ORIENTED_EDGE ( 'NONE', *, *, #15703, .F. ) ;
#7703=DIRECTION ( 'NONE',  ( 1.000000000000000000, 0.000000000000000000, -0.000000000000000000 ) ) ;
#7705=VERTEX_POINT ( 'NONE', #1360 ) ;
#7709=DIRECTION ( 'NONE',  ( -1.000000000000000000, -0.000000000000000000, -0.000000000000000000 ) ) ;
#7710=ORIENTED_EDGE ( 'NONE', *, *, #5047, .T. ) ;
#7717=ORIENTED_EDGE ( 'NONE', *, *, #6412, .T. ) ;
#7730=DIRECTION ( 'NONE',  ( 0.000000000000000000, 0.000000000000000000, -1.000000000000000000 ) ) ;
#7731=DIRECTION ( 'NONE',  ( -1.000000000000000000, -4.124608743189000987E-16, 0.000000000000000000 ) ) ;
#7733=DIRECTION ( 'NONE',  ( -0.000000000000000000, -0.000000000000000000, -1.000000000000000000 ) ) ;
#7736=DIRECTION ( 'NONE',  ( 1.000000000000000000, 0.000000000000000000, 0.000000000000000000 ) ) ;
#7738=EDGE_LOOP ( 'NONE', ( #12865, #6763, #9341, #5920, #8463 ) ) ;
#7758=CARTESIAN_POINT ( 'NONE',  ( -76.11074570696128205, 61.85979623000802974, -25.83329931759948295 ) ) ;
#7763=EDGE_CURVE ( 'NONE', #18214, #7705, #1288, .T. ) ;
#7765=B_SPLINE_CURVE_WITH_KNOTS ( 'NONE', 3,
 ( #6252, #16084, #11048, #18060 ),
 .UNSPECIFIED., .F., .F.,
 ( 4, 4 ),
 ( 0.000000000000000000, 0.002699315152504171492 ),
 .UNSPECIFIED. ) ;
#7769=EDGE_CURVE ( 'NONE', #4352, #11429, #18186, .T. ) ;
#7775=PLANE ( 'NONE',  #4866 ) ;
#7786=CARTESIAN_POINT ( 'NONE',  ( -70.71978124295696944, -141.5628872026273086, 18.23991632971911869 ) ) ;
#7798=ORIENTED_EDGE ( 'NONE', *, *, #15088, .T. ) ;
#7802=ORIENTED_EDGE ( 'NONE', *, *, #924, .T. ) ;
#7803=AXIS2_PLACEMENT_3D ( 'NONE', #10229, #14612, #8844 ) ;
#7805=CARTESIAN_POINT ( 'NONE',  ( -123.4618227840623632, -151.5628872026273086, 57.00000000000000000 ) ) ;
#7837=VECTOR ( 'NONE', #670, 1000.000000000000000 ) ;
#7841=ADVANCED_FACE ( 'NONE', ( #10983 ), #16669, .T. ) ;
#7855=CARTESIAN_POINT ( 'NONE',  ( -74.24049782422095234, 60.39151088118022415, -23.22272012184626178 ) ) ;
#7860=CARTESIAN_POINT ( 'NONE',  ( -92.59262256747319952, 50.58224449241410525, 35.00000000000000000 ) ) ;
#7864=ORIENTED_EDGE ( 'NONE', *, *, #9489, .T. ) ;
#7865=AXIS2_PLACEMENT_3D ( 'NONE', #10269, #15972, #2903 ) ;
#7868=FACE_OUTER_BOUND ( 'NONE', #14090, .T. ) ;
#7901=DIRECTION ( 'NONE',  ( 0.000000000000000000, 0.000000000000000000, 1.000000000000000000 ) ) ;
#7906=VERTEX_POINT ( 'NONE', #8643 ) ;
#7917=VECTOR ( 'NONE', #5410, 1000.000000000000000 ) ;
#7920=CARTESIAN_POINT ( 'NONE',  ( -83.12361985383350316, 84.22855780814606419, 37.50000000000000000 ) ) ;
#7925=CARTESIAN_POINT ( 'NONE',  ( 2.371465054068948142, 0.7538881668847053907, 50.31856894691938464 ) ) ;
#7927=DIRECTION ( 'NONE',  ( 0.000000000000000000, -0.000000000000000000, -1.000000000000000000 ) ) ;
#7933=( NAMED_UNIT ( * ) SI_UNIT ( $, .STERADIAN. ) SOLID_ANGLE_UNIT ( ) );
#7937=LINE ( 'NONE', #10729, #8804 ) ;
#7938=DIRECTION ( 'NONE',  ( 1.000000000000000000, 0.000000000000000000, 0.000000000000000000 ) ) ;
#7948=CARTESIAN_POINT ( 'NONE',  ( -67.59262256747315689, 129.5689604715732912, 15.00000000000005862 ) ) ;
#7964=DIRECTION ( 'NONE',  ( -1.000000000000000000, -0.000000000000000000, -0.000000000000000000 ) ) ;
#7965=CARTESIAN_POINT ( 'NONE',  ( 95.45835937779683888, -32.62665103886256190, -7.000000000000010658 ) ) ;
#7983=PLANE ( 'NONE',  #1054 ) ;
#7988=CARTESIAN_POINT ( 'NONE',  ( -74.87319944600693589, 107.5944659956890632, -23.67920958164899048 ) ) ;
#8001=VERTEX_POINT ( 'NONE', #10132 ) ;
#8005=DIRECTION ( 'NONE',  ( -0.000000000000000000, -0.000000000000000000, -1.000000000000000000 ) ) ;
#8009=EDGE_CURVE ( 'NONE', #299, #293, #1893, .T. ) ;
#8013=CARTESIAN_POINT ( 'NONE',  ( -64.09025127992791226, 117.8748711238780373, 35.00000000000000000 ) ) ;
#8033=EDGE_LOOP ( 'NONE', ( #4471, #330, #3550, #2997, #15851 ) ) ;
#8037=VECTOR ( 'NONE', #17914, 1000.000000000000000 ) ;
#8038=VERTEX_POINT ( 'NONE', #492 ) ;
#8049=CARTESIAN_POINT ( 'NONE',  ( 103.5381772159376084, 0.000000000000000000, 57.00000000000000000 ) ) ;
#8063=CIRCLE ( 'NONE', #892, 20.99999999999999645 ) ;
#8067=EDGE_LOOP ( 'NONE', ( #707, #12294, #5255, #6099, #15217, #12262 ) ) ;
#8070=VERTEX_POINT ( 'NONE', #16185 ) ;
#8083=CARTESIAN_POINT ( 'NONE',  ( -75.55027201341330567, 107.0628432229694340, -24.42475462179574919 ) ) ;
#8094=ORIENTED_EDGE ( 'NONE', *, *, #16008, .T. ) ;
#8097=CYLINDRICAL_SURFACE ( 'NONE', #18011, 85.91469608272775815 ) ;
#8098=PLANE ( 'NONE',  #7296 ) ;
#8106=LINE ( 'NONE', #5014, #8730 ) ;
#8119=ORIENTED_EDGE ( 'NONE', *, *, #13726, .F. ) ;
#8128=CARTESIAN_POINT ( 'NONE',  ( -64.09025127992791226, 117.8748711238780373, 35.00000000000000000 ) ) ;
#8148=EDGE_CURVE ( 'NONE', #9163, #1951, #15456, .T. ) ;
#8151=CARTESIAN_POINT ( 'NONE',  ( 124.5381772159375942, -151.5628872026272802, 36.00000000000001421 ) ) ;
#8156=DIRECTION ( 'NONE',  ( 1.000000000000000000, 4.675871521838984962E-16, -0.000000000000000000 ) ) ;
#8165=DIRECTION ( 'NONE',  ( -1.000000000000000000, -0.000000000000000000, -0.000000000000000000 ) ) ;
#8173=ORIENTED_EDGE ( 'NONE', *, *, #14863, .T. ) ;
#8174=CARTESIAN_POINT ( 'NONE',  ( -102.4618227840623774, -111.0842361345572158, -57.00000000000000000 ) ) ;
#8177=ORIENTED_EDGE ( 'NONE', *, *, #3089, .F. ) ;
#8180=DIRECTION ( 'NONE',  ( 4.675871521838985949E-16, -1.000000000000000000, -0.000000000000000000 ) ) ;
#8182=DIRECTION ( 'NONE',  ( -0.000000000000000000, -0.000000000000000000, 1.000000000000000000 ) ) ;
#8185=ORIENTED_EDGE ( 'NONE', *, *, #8363, .T. ) ;
#8187=CARTESIAN_POINT ( 'NONE',  ( -75.91366687898980103, 106.7636614011200891, -27.61062523460392981 ) ) ;
#8194=ORIENTED_EDGE ( 'NONE', *, *, #8775, .F. ) ;
#8196=CIRCLE ( 'NONE', #9748, 34.36884788726141693 ) ;
#8197=VECTOR ( 'NONE', #2472, 1000.000000000000114 ) ;
#8198=CIRCLE ( 'NONE', #14758, 85.91469608272775815 ) ;
#8200=CARTESIAN_POINT ( 'NONE',  ( -67.59262256747315689, 111.6514400295689313, -15.00000000000001066 ) ) ;
#8202=CARTESIAN_POINT ( 'NONE',  ( 49.38736944425944841, -141.5628872026273086, -57.00000000000000000 ) ) ;
#8203=DIRECTION ( 'NONE',  ( -0.000000000000000000, -0.000000000000000000, 1.000000000000000000 ) ) ;
#8205=FACE_OUTER_BOUND ( 'NONE', #16973, .T. ) ;
#8211=CARTESIAN_POINT ( 'NONE',  ( -21.28916685891738325, 36.54437923629615170, -35.57537618398750823 ) ) ;
#8219=DIRECTION ( 'NONE',  ( 4.675871521838985949E-16, -1.000000000000000000, -0.000000000000000000 ) ) ;
#8230=LINE ( 'NONE', #2709, #16820 ) ;
#8233=DIRECTION ( 'NONE',  ( 0.000000000000000000, 1.000000000000000000, 0.000000000000000000 ) ) ;
#8234=CARTESIAN_POINT ( 'NONE',  ( -67.59262256747315689, 129.5689604715732912, -15.00000000000001066 ) ) ;
#8239=EDGE_CURVE ( 'NONE', #2148, #17871, #6840, .T. ) ;
#8250=EDGE_CURVE ( 'NONE', #14911, #9679, #4850, .T. ) ;
#8251=ORIENTED_EDGE ( 'NONE', *, *, #1969, .T. ) ;
#8255=CARTESIAN_POINT ( 'NONE',  ( -66.63376473465912397, -19.34983604512935429, -3.000000000000000000 ) ) ;
#8260=ADVANCED_FACE ( 'NONE', ( #13963 ), #18261, .T. ) ;
#8261=CARTESIAN_POINT ( 'NONE',  ( -67.59262256747319952, 111.6514400295689171, 22.50837044127971254 ) ) ;
#8263=CARTESIAN_POINT ( 'NONE',  ( 5.233202738124664855, -111.0842361345572158, 57.00000000000000000 ) ) ;
#8265=DIRECTION ( 'NONE',  ( -0.000000000000000000, 0.000000000000000000, 1.000000000000000000 ) ) ;
#8268=DIRECTION ( 'NONE',  ( -1.000000000000000000, -0.000000000000000000, -0.000000000000000000 ) ) ;
#8271=VERTEX_POINT ( 'NONE', #17203 ) ;
#8272=EDGE_CURVE ( 'NONE', #9327, #8420, #4387, .T. ) ;
#8275=DIRECTION ( 'NONE',  ( 1.000000000000000000, 0.000000000000000000, 0.000000000000000000 ) ) ;
#8280=CARTESIAN_POINT ( 'NONE',  ( 15.23320273812466219, -15.06406080364910771, -54.10850799397452704 ) ) ;
#8285=CARTESIAN_POINT ( 'NONE',  ( 95.45835937779679625, 56.41207303426869402, 7.000000000000010658 ) ) ;
#8286=ORIENTED_EDGE ( 'NONE', *, *, #6780, .F. ) ;
#8288=LINE ( 'NONE', #11092, #2464 ) ;
#8290=CARTESIAN_POINT ( 'NONE',  ( -64.09025127992791226, 117.8748711238780373, -7.000000000000013323 ) ) ;
#8292=ORIENTED_EDGE ( 'NONE', *, *, #14508, .F. ) ;
#8303=CARTESIAN_POINT ( 'NONE',  ( -24.41997999089026550, 38.95069813737347886, -34.21586952458824982 ) ) ;
#8304=CARTESIAN_POINT ( 'NONE',  ( 3.080246995596566340, 23.75572429475707636, 41.96082232098843434 ) ) ;
#8317=LINE ( 'NONE', #9529, #1588 ) ;
#8318=CIRCLE ( 'NONE', #2942, 3.999999999999982681 ) ;
#8319=DIRECTION ( 'NONE',  ( 0.000000000000000000, 0.000000000000000000, 1.000000000000000000 ) ) ;
#8320=ORIENTED_EDGE ( 'NONE', *, *, #10923, .T. ) ;
#8321=CARTESIAN_POINT ( 'NONE',  ( -66.26485270048019061, 109.8219421365140249, -28.00000000000000000 ) ) ;
#8329=B_SPLINE_CURVE_WITH_KNOTS ( 'NONE', 3,
 ( #9866, #8280, #2858, #13898, #13990, #18103, #16771, #8369, #16672, #5460, #2759, #5356, #8465, #1263, #1445, #9776, #1170, #14176, #11370, #7069, #6779, #9680, #6868, #5558, #4158, #15390, #12781, #2579 ),
 .UNSPECIFIED., .F., .F.,
 ( 4, 2, 2, 2, 2, 2, 2, 2, 2, 2, 2, 2, 2, 4 ),
 ( 0.000000000000000000, 0.01281839044724412263, 0.02563678089448824526, 0.02884137850629928113, 0.03204597611811031699, 0.03845517134173238177, 0.05127356178897649747, 0.05768275701259856225, 0.06409195223622063398, 0.07691034268346474967, 0.08331953790708679364, 0.08652413551889782950, 0.08972873313070885148, 0.1025471235779529533 ),
 .UNSPECIFIED. ) ;
#8331=ORIENTED_EDGE ( 'NONE', *, *, #18075, .F. ) ;
#8338=CARTESIAN_POINT ( 'NONE',  ( -69.25739799065789271, 57.48797571754649738, -22.35917033480642502 ) ) ;
#8350=CARTESIAN_POINT ( 'NONE',  ( 95.45835937779679625, 56.41207303426869402, 3.000000000000000000 ) ) ;
#8352=ORIENTED_EDGE ( 'NONE', *, *, #16945, .F. ) ;
#8356=EDGE_CURVE ( 'NONE', #573, #18453, #1750, .T. ) ;
#8363=EDGE_CURVE ( 'NONE', #6958, #15269, #7286, .T. ) ;
#8368=ORIENTED_EDGE ( 'NONE', *, *, #116, .F. ) ;
#8369=CARTESIAN_POINT ( 'NONE',  ( 10.09019014590969654, 9.228091135629581387, -47.65272416155497837 ) ) ;
#8372=EDGE_CURVE ( 'NONE', #3309, #12209, #10545, .T. ) ;
#8382=CIRCLE ( 'NONE', #8680, 34.36884788726143114 ) ;
#8384=CARTESIAN_POINT ( 'NONE',  ( -100.4870060002411805, -151.5628872026273086, -18.23991632971910803 ) ) ;
#8414=CARTESIAN_POINT ( 'NONE',  ( -57.08002265617300708, 84.22855780814606419, 37.50000000000000000 ) ) ;
#8418=DIRECTION ( 'NONE',  ( 0.000000000000000000, -0.000000000000000000, -1.000000000000000000 ) ) ;
#8420=VERTEX_POINT ( 'NONE', #13007 ) ;
#8422=CIRCLE ( 'NONE', #337, 29.36884788726140627 ) ;
#8442=LINE ( 'NONE', #12562, #13436 ) ;
#8447=CARTESIAN_POINT ( 'NONE',  ( 0.000000000000000000, 0.000000000000000000, 3.000000000000000000 ) ) ;
#8449=CIRCLE ( 'NONE', #6319, 85.91469608272775815 ) ;
#8452=EDGE_CURVE ( 'NONE', #10991, #8271, #7456, .T. ) ;
#8461=CARTESIAN_POINT ( 'NONE',  ( 15.23320273812466041, -19.34983604512935429, 57.00000000000000000 ) ) ;
#8463=ORIENTED_EDGE ( 'NONE', *, *, #15789, .F. ) ;
#8465=CARTESIAN_POINT ( 'NONE',  ( 3.062581012969010974, 23.78654787968694961, -41.94750742838608915 ) ) ;
#8473=ADVANCED_FACE ( 'NONE', ( #17543 ), #8097, .F. ) ;
#8476=VERTEX_POINT ( 'NONE', #3605 ) ;
#8480=DIRECTION ( 'NONE',  ( 0.000000000000000000, 0.000000000000000000, -1.000000000000000000 ) ) ;
#8504=CARTESIAN_POINT ( 'NONE',  ( -29.49754210169703939, 42.18689076489602741, -32.29756042961390960 ) ) ;
#8511=CARTESIAN_POINT ( 'NONE',  ( -123.4618227840623632, -111.0842361345572158, 7.000000000000013323 ) ) ;
#8517=EDGE_CURVE ( 'NONE', #7155, #16713, #5299, .T. ) ;
#8518=CYLINDRICAL_SURFACE ( 'NONE', #12364, 26.04359719766049253 ) ;
#8521=CARTESIAN_POINT ( 'NONE',  ( -66.71236600666622962, 111.9737865874585481, -24.23198523837357143 ) ) ;
#8522=CARTESIAN_POINT ( 'NONE',  ( -75.31304609867017064, 61.20467279731714427, 24.11916851373873882 ) ) ;
#8524=VERTEX_POINT ( 'NONE', #13816 ) ;
#8526=CARTESIAN_POINT ( 'NONE',  ( -64.09025127992788384, 50.58224449241410525, 35.00000000000000000 ) ) ;
#8529=LINE ( 'NONE', #17208, #1083 ) ;
#8530=VECTOR ( 'NONE', #6751, 1000.000000000000000 ) ;
#8537=VERTEX_POINT ( 'NONE', #9325 ) ;
#8560=CARTESIAN_POINT ( 'NONE',  ( 95.45835937779682467, 4.463510241361116170E-14, -3.000000000000000000 ) ) ;
#8563=LINE ( 'NONE', #18287, #14382 ) ;
#8570=CARTESIAN_POINT ( 'NONE',  ( 79.02261728059691848, -151.5628872026273086, 57.00000000000000000 ) ) ;
#8572=EDGE_CURVE ( 'NONE', #10176, #8070, #5006, .T. ) ;
#8590=EDGE_CURVE ( 'NONE', #2581, #6749, #11270, .T. ) ;
#8595=CARTESIAN_POINT ( 'NONE',  ( -44.49764538373973721, 84.22855780814606419, 25.00000000000000355 ) ) ;
#8601=CARTESIAN_POINT ( 'NONE',  ( -64.09025127992788384, 50.58224449241410525, 35.00000000000000000 ) ) ;
#8610=CARTESIAN_POINT ( 'NONE',  ( -38.40244272411881354, 55.35140561506842261, 23.53852893732882379 ) ) ;
#8624=DIRECTION ( 'NONE',  ( -0.000000000000000000, -0.000000000000000000, -1.000000000000000000 ) ) ;
#8629=LINE ( 'NONE', #12846, #10497 ) ;
#8638=ORIENTED_EDGE ( 'NONE', *, *, #687, .F. ) ;
#8643=CARTESIAN_POINT ( 'NONE',  ( -67.59262256747315689, 117.8748711238780373, -15.00000000000001066 ) ) ;
#8646=VERTEX_POINT ( 'NONE', #1293 ) ;
#8650=VERTEX_POINT ( 'NONE', #12799 ) ;
#8652=ORIENTED_EDGE ( 'NONE', *, *, #11095, .T. ) ;
#8657=AXIS2_PLACEMENT_3D ( 'NONE', #4177, #18018, #16900 ) ;
#8672=ORIENTED_EDGE ( 'NONE', *, *, #8942, .T. ) ;
#8675=DIRECTION ( 'NONE',  ( 0.000000000000000000, 1.000000000000000000, 0.000000000000000000 ) ) ;
#8680=AXIS2_PLACEMENT_3D ( 'NONE', #5035, #16540, #2047 ) ;
#8685=CARTESIAN_POINT ( 'NONE',  ( -66.22475908702843128, 112.1374203547857036, -25.60634877502412721 ) ) ;
#8694=DIRECTION ( 'NONE',  ( 2.062304371594500494E-16, -1.000000000000000000, 0.000000000000000000 ) ) ;
#8695=DIRECTION ( 'NONE',  ( -1.000000000000000000, -0.000000000000000000, -0.000000000000000000 ) ) ;
#8696=ORIENTED_EDGE ( 'NONE', *, *, #17385, .T. ) ;
#8701=LINE ( 'NONE', #17118, #11070 ) ;
#8722=ORIENTED_EDGE ( 'NONE', *, *, #8775, .T. ) ;
#8730=VECTOR ( 'NONE', #9333, 1000.000000000000000 ) ;
#8731=AXIS2_PLACEMENT_3D ( 'NONE', #4751, #6242, #476 ) ;
#8733=EDGE_CURVE ( 'NONE', #5426, #16629, #8422, .T. ) ;
#8735=EDGE_LOOP ( 'NONE', ( #12133, #3488, #16447, #4719 ) ) ;
#8736=AXIS2_PLACEMENT_3D ( 'NONE', #17899, #3502, #2008 ) ;
#8737=CARTESIAN_POINT ( 'NONE',  ( -67.59262256747315689, 56.80567558672318285, 37.50000000000000000 ) ) ;
#8748=DIRECTION ( 'NONE',  ( -0.000000000000000000, -0.000000000000000000, 1.000000000000000000 ) ) ;
#8752=AXIS2_PLACEMENT_3D ( 'NONE', #3864, #9571, #13892 ) ;
#8757=CARTESIAN_POINT ( 'NONE',  ( 0.000000000000000000, 0.000000000000000000, 35.00000000000000000 ) ) ;
#8773=PLANE ( 'NONE',  #12642 ) ;
#8775=EDGE_CURVE ( 'NONE', #3955, #4742, #5928, .T. ) ;
#8779=ORIENTED_EDGE ( 'NONE', *, *, #2509, .T. ) ;
#8804=VECTOR ( 'NONE', #16425, 1000.000000000000000 ) ;
#8806=CIRCLE ( 'NONE', #4331, 3.999999999999989786 ) ;
#8814=PLANE ( 'NONE',  #17081 ) ;
#8821=AXIS2_PLACEMENT_3D ( 'NONE', #14188, #6790, #8480 ) ;
#8826=DIRECTION ( 'NONE',  ( -1.000000000000000000, 0.000000000000000000, 0.000000000000000000 ) ) ;
#8841=EDGE_CURVE ( 'NONE', #3501, #2330, #17807, .T. ) ;
#8844=DIRECTION ( 'NONE',  ( 0.000000000000000000, -0.000000000000000000, -1.000000000000000000 ) ) ;
#8849=VERTEX_POINT ( 'NONE', #6390 ) ;
#8861=ORIENTED_EDGE ( 'NONE', *, *, #14754, .T. ) ;
#8872=CARTESIAN_POINT ( 'NONE',  ( -46.03642545851251100, 84.22855780814606419, -47.49999999999999289 ) ) ;
#8897=DIRECTION ( 'NONE',  ( 0.000000000000000000, 0.000000000000000000, 1.000000000000000000 ) ) ;
#8898=LINE ( 'NONE', #11800, #10215 ) ;
#8900=DIRECTION ( 'NONE',  ( 1.000000000000000000, 0.000000000000000000, 0.000000000000000000 ) ) ;
#8905=CARTESIAN_POINT ( 'NONE',  ( -67.59262256747317110, 57.88796029049329661, 26.35917033480641436 ) ) ;
#8922=CARTESIAN_POINT ( 'NONE',  ( 105.4583593777968105, 56.41207303426870112, 7.000000000000010658 ) ) ;
#8929=ADVANCED_FACE ( 'NONE', ( #9303 ), #5707, .F. ) ;
#8934=EDGE_CURVE ( 'NONE', #1708, #11504, #12611, .T. ) ;
#8940=CARTESIAN_POINT ( 'NONE',  ( -127.5926225674731995, 110.5691553257988460, 22.35917033480641791 ) ) ;
#8942=EDGE_CURVE ( 'NONE', #6285, #4169, #8329, .T. ) ;
#8943=CARTESIAN_POINT ( 'NONE',  ( -36.44155368744861079, 56.74635804676025685, 0.000000000000000000 ) ) ;
#8944=AXIS2_PLACEMENT_3D ( 'NONE', #2495, #8203, #2788 ) ;
#8961=DIRECTION ( 'NONE',  ( 1.000000000000000000, 0.000000000000000000, 0.000000000000000000 ) ) ;
#8966=FACE_OUTER_BOUND ( 'NONE', #523, .T. ) ;
#8973=CARTESIAN_POINT ( 'NONE',  ( -64.09025127992788384, 59.14618053571278722, 35.00000000000000000 ) ) ;
#8977=CIRCLE ( 'NONE', #11072, 3.999999999999989786 ) ;
#8991=ORIENTED_EDGE ( 'NONE', *, *, #6495, .T. ) ;
#8997=EDGE_CURVE ( 'NONE', #11177, #15813, #8563, .T. ) ;
#9008=ORIENTED_EDGE ( 'NONE', *, *, #14548, .F. ) ;
#9041=DIRECTION ( 'NONE',  ( -1.000000000000000000, -0.000000000000000000, -0.000000000000000000 ) ) ;
#9044=PLANE ( 'NONE',  #15826 ) ;
#9046=ORIENTED_EDGE ( 'NONE', *, *, #1173, .F. ) ;
#9047=ORIENTED_EDGE ( 'NONE', *, *, #16664, .T. ) ;
#9052=AXIS2_PLACEMENT_3D ( 'NONE', #10379, #3182, #11794 ) ;
#9058=FACE_OUTER_BOUND ( 'NONE', #1133, .T. ) ;
#9061=LINE ( 'NONE', #1947, #173 ) ;
#9062=FACE_OUTER_BOUND ( 'NONE', #3195, .T. ) ;
#9068=ORIENTED_EDGE ( 'NONE', *, *, #16236, .T. ) ;
#9075=AXIS2_PLACEMENT_3D ( 'NONE', #6456, #3557, #16463 ) ;
#9081=CARTESIAN_POINT ( 'NONE',  ( 103.5381772159376084, -151.5628872026272802, -36.00000000000000000 ) ) ;
#9086=CARTESIAN_POINT ( 'NONE',  ( -42.13578017738746695, 48.33287759230859137, -28.43492242011098625 ) ) ;
#9098=DIRECTION ( 'NONE',  ( -1.000000000000000000, -0.000000000000000000, -0.000000000000000000 ) ) ;
#9110=AXIS2_PLACEMENT_3D ( 'NONE', #7434, #510, #15861 ) ;
#9111=ORIENTED_EDGE ( 'NONE', *, *, #4936, .T. ) ;
#9128=VERTEX_POINT ( 'NONE', #7965 ) ;
#9129=CARTESIAN_POINT ( 'NONE',  ( 124.5381772159375942, -111.0842361345572158, 36.00000000000001421 ) ) ;
#9132=VECTOR ( 'NONE', #188, 1000.000000000000000 ) ;
#9139=ORIENTED_EDGE ( 'NONE', *, *, #16942, .F. ) ;
#9141=DIRECTION ( 'NONE',  ( 1.119176436114069332E-16, -1.000000000000000000, -0.000000000000000000 ) ) ;
#9153=DIRECTION ( 'NONE',  ( 0.000000000000000000, 0.000000000000000000, 1.000000000000000000 ) ) ;
#9155=ORIENTED_EDGE ( 'NONE', *, *, #10409, .F. ) ;
#9163=VERTEX_POINT ( 'NONE', #4228 ) ;
#9170=LINE ( 'NONE', #14856, #15064 ) ;
#9185=ORIENTED_EDGE ( 'NONE', *, *, #16366, .T. ) ;
#9190=CARTESIAN_POINT ( 'NONE',  ( 5.233202738124664855, -46.83756720124470263, 57.00000000000000000 ) ) ;
#9193=PLANE ( 'NONE',  #1018 ) ;
#9196=CARTESIAN_POINT ( 'NONE',  ( -70.06856178257680767, 110.5691553257988460, -22.35917033480641791 ) ) ;
#9209=ORIENTED_EDGE ( 'NONE', *, *, #3882, .F. ) ;
#9212=ORIENTED_EDGE ( 'NONE', *, *, #17178, .T. ) ;
#9223=VERTEX_POINT ( 'NONE', #13772 ) ;
#9228=CARTESIAN_POINT ( 'NONE',  ( 5.233202738124664855, -19.34983604512936495, 54.79921157549230770 ) ) ;
#9229=AXIS2_PLACEMENT_3D ( 'NONE', #11744, #11646, #4626 ) ;
#9230=CARTESIAN_POINT ( 'NONE',  ( -57.08002265617300708, 84.22855780814606419, -7.000000000000013323 ) ) ;
#9236=ORIENTED_EDGE ( 'NONE', *, *, #15769, .F. ) ;
#9256=CARTESIAN_POINT ( 'NONE',  ( -70.85175816390371040, -141.5628872026273086, -57.00000000000000000 ) ) ;
#9257=CARTESIAN_POINT ( 'NONE',  ( -194.4437806548868934, -151.5628872026273086, -18.23991632971910803 ) ) ;
#9262=CARTESIAN_POINT ( 'NONE',  ( -74.87388236440091305, 60.86317103097213277, -23.67979665430766190 ) ) ;
#9263=AXIS2_PLACEMENT_3D ( 'NONE', #14591, #1773, #6069 ) ;
#9268=EDGE_CURVE ( 'NONE', #14872, #293, #14513, .T. ) ;
#9273=EDGE_CURVE ( 'NONE', #15127, #4073, #1691, .T. ) ;
#9276=DIRECTION ( 'NONE',  ( 0.000000000000000000, 0.000000000000000000, 1.000000000000000000 ) ) ;
#9289=ORIENTED_EDGE ( 'NONE', *, *, #16336, .T. ) ;
#9291=EDGE_CURVE ( 'NONE', #1462, #16981, #8898, .T. ) ;
#9294=AXIS2_PLACEMENT_3D ( 'NONE', #10645, #15123, #7730 ) ;
#9303=FACE_OUTER_BOUND ( 'NONE', #2062, .T. ) ;
#9317=ORIENTED_EDGE ( 'NONE', *, *, #9609, .T. ) ;
#9318=VERTEX_POINT ( 'NONE', #13202 ) ;
#9325=CARTESIAN_POINT ( 'NONE',  ( -70.85175816390371040, -141.5628872026273086, 57.00000000000000000 ) ) ;
#9327=VERTEX_POINT ( 'NONE', #205 ) ;
#9329=CARTESIAN_POINT ( 'NONE',  ( -92.59262256747321373, 117.8748711238780373, -35.00000000000000000 ) ) ;
#9333=DIRECTION ( 'NONE',  ( -0.000000000000000000, -0.000000000000000000, -1.000000000000000000 ) ) ;
#9337=ORIENTED_EDGE ( 'NONE', *, *, #4046, .T. ) ;
#9341=ORIENTED_EDGE ( 'NONE', *, *, #11337, .T. ) ;
#9344=VECTOR ( 'NONE', #15937, 1000.000000000000000 ) ;
#9347=DIRECTION ( 'NONE',  ( -1.000000000000000000, -0.000000000000000000, -0.000000000000000000 ) ) ;
#9349=CARTESIAN_POINT ( 'NONE',  ( -67.59262256747317110, 61.53592931583062153, -28.00000000000000355 ) ) ;
#9355=EDGE_CURVE ( 'NONE', #6374, #15744, #8629, .T. ) ;
#9356=LINE ( 'NONE', #843, #5174 ) ;
#9371=DIRECTION ( 'NONE',  ( -0.000000000000000000, -0.000000000000000000, -1.000000000000000000 ) ) ;
#9372=CARTESIAN_POINT ( 'NONE',  ( -102.4618227840623774, -111.0842361345572158, -57.00000000000000000 ) ) ;
#9385=ADVANCED_FACE ( 'NONE', ( #10362 ), #1888, .F. ) ;
#9388=AXIS2_PLACEMENT_3D ( 'NONE', #9462, #6657, #3939 ) ;
#9390=EDGE_CURVE ( 'NONE', #2581, #18214, #13033, .T. ) ;
#9391=ADVANCED_FACE ( 'NONE', ( #3100 ), #8814, .F. ) ;
#9402=AXIS2_PLACEMENT_3D ( 'NONE', #2139, #17941, #17563 ) ;
#9404=CARTESIAN_POINT ( 'NONE',  ( -92.59262256747319952, 57.88796029049329661, 26.35917033480641436 ) ) ;
#9408=LINE ( 'NONE', #880, #11696 ) ;
#9412=AXIS2_PLACEMENT_3D ( 'NONE', #14445, #10048, #11549 ) ;
#9421=CARTESIAN_POINT ( 'NONE',  ( 124.5381772159375942, -111.0842361345572158, 57.00000000000000000 ) ) ;
#9423=ORIENTED_EDGE ( 'NONE', *, *, #11329, .F. ) ;
#9424=CARTESIAN_POINT ( 'NONE',  ( -75.72335493167709330, 106.9211863004614997, -28.00000000000000355 ) ) ;
#9425=CARTESIAN_POINT ( 'NONE',  ( -4.730921629999971678, 17.21234141005219698, 44.69891962609317204 ) ) ;
#9433=ORIENTED_EDGE ( 'NONE', *, *, #16448, .F. ) ;
#9436=ORIENTED_EDGE ( 'NONE', *, *, #12596, .F. ) ;
#9439=VERTEX_POINT ( 'NONE', #552 ) ;
#9453=ORIENTED_EDGE ( 'NONE', *, *, #468, .F. ) ;
#9458=ORIENTED_EDGE ( 'NONE', *, *, #17048, .F. ) ;
#9459=ORIENTED_EDGE ( 'NONE', *, *, #13268, .F. ) ;
#9462=CARTESIAN_POINT ( 'NONE',  ( -127.5926225674731711, 57.88796029049329661, -26.35917033480641436 ) ) ;
#9477=CARTESIAN_POINT ( 'NONE',  ( -127.5926225674731711, 57.88796029049329661, -30.35917033480640370 ) ) ;
#9486=DIRECTION ( 'NONE',  ( 0.000000000000000000, 0.000000000000000000, 1.000000000000000000 ) ) ;
#9489=EDGE_CURVE ( 'NONE', #8001, #6374, #14397, .T. ) ;
#9491=CARTESIAN_POINT ( 'NONE',  ( -67.59262256747319952, 106.8071537307723133, 25.00000000000000355 ) ) ;
#9499=ADVANCED_FACE ( 'NONE', ( #10670 ), #13298, .F. ) ;
#9502=DIRECTION ( 'NONE',  ( -1.000000000000000000, 0.000000000000000000, -9.912705577010330480E-16 ) ) ;
#9503=ORIENTED_EDGE ( 'NONE', *, *, #5271, .T. ) ;
#9508=DIRECTION ( 'NONE',  ( 0.000000000000000000, 0.000000000000000000, -1.000000000000000000 ) ) ;
#9514=CARTESIAN_POINT ( 'NONE',  ( -18.61292065092662185, 46.98476669316325172, 29.30995736292643628 ) ) ;
#9519=ADVANCED_FACE ( 'NONE', ( #13471 ), #6343, .T. ) ;
#9527=ORIENTED_EDGE ( 'NONE', *, *, #16448, .T. ) ;
#9529=CARTESIAN_POINT ( 'NONE',  ( -100.4870060002411805, -151.5628872026273086, -57.00000000000000000 ) ) ;
#9530=CARTESIAN_POINT ( 'NONE',  ( -67.15995696847650720, 60.73698500726539606, -28.00000000000000355 ) ) ;
#9533=CARTESIAN_POINT ( 'NONE',  ( -70.71978124295696944, -141.5628872026273086, 5.204170427930421283E-15 ) ) ;
#9545=ORIENTED_EDGE ( 'NONE', *, *, #4926, .F. ) ;
#9547=CARTESIAN_POINT ( 'NONE',  ( 103.5381772159376084, -111.0842361345572158, 57.00000000000000000 ) ) ;
#9555=VERTEX_POINT ( 'NONE', #15439 ) ;
#9559=VERTEX_POINT ( 'NONE', #6737 ) ;
#9561=PLANE ( 'NONE',  #17689 ) ;
#9566=CIRCLE ( 'NONE', #15242, 3.999999999999989786 ) ;
#9568=ORIENTED_EDGE ( 'NONE', *, *, #727, .F. ) ;
#9571=DIRECTION ( 'NONE',  ( 0.000000000000000000, -1.000000000000000000, 0.000000000000000000 ) ) ;
#9577=ORIENTED_EDGE ( 'NONE', *, *, #416, .F. ) ;
#9580=DIRECTION ( 'NONE',  ( 1.000000000000000000, 0.000000000000000000, 0.000000000000000000 ) ) ;
#9584=CARTESIAN_POINT ( 'NONE',  ( -70.06856178257680767, 110.5691553257988460, -22.35917033480641791 ) ) ;
#9590=ORIENTED_EDGE ( 'NONE', *, *, #11566, .F. ) ;
#9591=VECTOR ( 'NONE', #14351, 1000.000000000000000 ) ;
#9598=FACE_OUTER_BOUND ( 'NONE', #6818, .T. ) ;
#9601=DIRECTION ( 'NONE',  ( -1.000000000000000000, 0.000000000000000000, 0.000000000000000000 ) ) ;
#9607=CARTESIAN_POINT ( 'NONE',  ( -4.030484272568896742, 33.41412046829307059, 37.23164655599730821 ) ) ;
#9609=EDGE_CURVE ( 'NONE', #10351, #16485, #8449, .T. ) ;
#9611=VECTOR ( 'NONE', #4395, 1000.000000000000000 ) ;
#9615=CARTESIAN_POINT ( 'NONE',  ( -57.08002265617300708, 84.22855780814606419, 28.00000000000000355 ) ) ;
#9621=EDGE_CURVE ( 'NONE', #4482, #13472, #2714, .T. ) ;
#9622=DIRECTION ( 'NONE',  ( 4.124608743189000987E-16, -1.000000000000000000, 0.000000000000000000 ) ) ;
#9623=ORIENTED_EDGE ( 'NONE', *, *, #9851, .T. ) ;
#9624=AXIS2_PLACEMENT_3D ( 'NONE', #12026, #12310, #10805 ) ;
#9625=VECTOR ( 'NONE', #15342, 1000.000000000000000 ) ;
#9627=CARTESIAN_POINT ( 'NONE',  ( -66.56181127008836995, 56.43195750230852070, 24.56257327959996317 ) ) ;
#9633=LINE ( 'NONE', #8234, #11224 ) ;
#9638=CONICAL_SURFACE ( 'NONE', #13232, 3.999999999999989786, 1.029744258676652091 ) ;
#9644=CARTESIAN_POINT ( 'NONE',  ( 103.5381772159376084, -151.5628872026272802, -36.00000000000000000 ) ) ;
#9651=CARTESIAN_POINT ( 'NONE',  ( -123.4618227840623632, -111.0842361345572158, 18.23991632971911869 ) ) ;
#9652=DIRECTION ( 'NONE',  ( -0.000000000000000000, -0.000000000000000000, -1.000000000000000000 ) ) ;
#9656=AXIS2_PLACEMENT_3D ( 'NONE', #3820, #12243, #2042 ) ;
#9658=ORIENTED_EDGE ( 'NONE', *, *, #5843, .T. ) ;
#9677=ORIENTED_EDGE ( 'NONE', *, *, #3858, .T. ) ;
#9678=SHAPE_DEFINITION_REPRESENTATION ( #6699, #17553 ) ;
#9679=VERTEX_POINT ( 'NONE', #3923 ) ;
#9680=CARTESIAN_POINT ( 'NONE',  ( -21.14627411319134254, 48.72449396156541468, -28.16502384431897710 ) ) ;
#9691=EDGE_LOOP ( 'NONE', ( #4975, #2188, #13311, #14063, #7339, #9762 ) ) ;
#9694=VECTOR ( 'NONE', #2359, 1000.000000000000000 ) ;
#9695=CARTESIAN_POINT ( 'NONE',  ( -66.51107682098671603, 56.41472097771080030, -24.67867649519316586 ) ) ;
#9697=VECTOR ( 'NONE', #52, 1000.000000000000000 ) ;
#9712=CARTESIAN_POINT ( 'NONE',  ( -5.674266893243433252, 18.91634531463802205, -44.04015471320351338 ) ) ;
#9713=CARTESIAN_POINT ( 'NONE',  ( 7.760541235713054320, 14.88095002529105493, 45.61112162941545023 ) ) ;
#9720=EDGE_CURVE ( 'NONE', #7155, #16062, #3829, .T. ) ;
#9722=CARTESIAN_POINT ( 'NONE',  ( -194.4437806548868934, -151.5628872026273086, -18.23991632971910803 ) ) ;
#9728=ADVANCED_FACE ( 'NONE', ( #16834 ), #5877, .F. ) ;
#9732=CARTESIAN_POINT ( 'NONE',  ( -75.58239991587453233, 61.41969864223252529, 24.46191329895506783 ) ) ;
#9735=DIRECTION ( 'NONE',  ( -4.124608743189000987E-16, 1.000000000000000000, 0.000000000000000000 ) ) ;
#9737=DIRECTION ( 'NONE',  ( -1.000000000000000000, -0.000000000000000000, -0.000000000000000000 ) ) ;
#9741=DIRECTION ( 'NONE',  ( 1.000000000000000000, 0.000000000000000000, 0.000000000000000000 ) ) ;
#9748=AXIS2_PLACEMENT_3D ( 'NONE', #10779, #14977, #3764 ) ;
#9749=ORIENTED_EDGE ( 'NONE', *, *, #18430, .T. ) ;
#9758=CARTESIAN_POINT ( 'NONE',  ( -57.08002265617300708, 84.22855780814606419, 28.00000000000000355 ) ) ;
#9762=ORIENTED_EDGE ( 'NONE', *, *, #934, .F. ) ;
#9765=DIRECTION ( 'NONE',  ( 1.000000000000000000, 0.000000000000000000, 0.000000000000000000 ) ) ;
#9773=DIRECTION ( 'NONE',  ( -1.000000000000000000, -0.000000000000000000, -0.000000000000000000 ) ) ;
#9776=CARTESIAN_POINT ( 'NONE',  ( -4.069817365965976208, 33.48920034010672708, -37.19988592485734102 ) ) ;
#9778=ORIENTED_EDGE ( 'NONE', *, *, #13046, .T. ) ;
#9779=LINE ( 'NONE', #1092, #12285 ) ;
#9780=DIRECTION ( 'NONE',  ( -0.000000000000000000, -0.000000000000000000, -1.000000000000000000 ) ) ;
#9783=CARTESIAN_POINT ( 'NONE',  ( -72.05036370780659638, 109.4994693637201664, -22.49689322592065466 ) ) ;
#9792=DIRECTION ( 'NONE',  ( 1.000000000000000000, 0.000000000000000000, 0.000000000000000000 ) ) ;
#9796=CARTESIAN_POINT ( 'NONE',  ( -42.13624723507101066, 48.33286343412846975, 28.43491036791323623 ) ) ;
#9801=LINE ( 'NONE', #7607, #1084 ) ;
#9802=CARTESIAN_POINT ( 'NONE',  ( -74.59024599270496481, 107.8080920662734314, 23.45507754830875413 ) ) ;
#9804=CARTESIAN_POINT ( 'NONE',  ( 3.412248078327399625, -3.148451073394814337, -51.39674937110251562 ) ) ;
#9807=CARTESIAN_POINT ( 'NONE',  ( 95.45835937779683888, -32.62665103886256190, 3.000000000000000000 ) ) ;
#9809=LINE ( 'NONE', #8511, #15849 ) ;
#9813=DIRECTION ( 'NONE',  ( 0.000000000000000000, 0.000000000000000000, 1.000000000000000000 ) ) ;
#9824=CARTESIAN_POINT ( 'NONE',  ( 105.4583593777967963, -32.62665103886256190, 7.000000000000010658 ) ) ;
#9835=EDGE_CURVE ( 'NONE', #18083, #11856, #6628, .T. ) ;
#9851=EDGE_CURVE ( 'NONE', #13685, #9953, #10824, .T. ) ;
#9852=EDGE_CURVE ( 'NONE', #6748, #9223, #18001, .T. ) ;
#9866=CARTESIAN_POINT ( 'NONE',  ( 15.23320273812466041, -19.34983604512934363, -54.79921157549233612 ) ) ;
#9873=EDGE_LOOP ( 'NONE', ( #7516, #16278, #12206, #10320, #2865, #14788, #6541 ) ) ;
#9877=EDGE_CURVE ( 'NONE', #748, #2148, #10510, .T. ) ;
#9878=CIRCLE ( 'NONE', #9263, 170.8515291679562154 ) ;
#9886=AXIS2_PLACEMENT_3D ( 'NONE', #12055, #6228, #14759 ) ;
#9893=CARTESIAN_POINT ( 'NONE',  ( -9.128655484568604095, 23.76631003692282462, 41.91653839390071568 ) ) ;
#9895=ORIENTED_EDGE ( 'NONE', *, *, #16947, .T. ) ;
#9909=ORIENTED_EDGE ( 'NONE', *, *, #15769, .T. ) ;
#9911=ADVANCED_FACE ( 'NONE', ( #9062 ), #7558, .F. ) ;
#9918=CARTESIAN_POINT ( 'NONE',  ( -66.16666462472026922, 110.5025503192935474, -27.99999999999999289 ) ) ;
#9924=ORIENTED_EDGE ( 'NONE', *, *, #13046, .F. ) ;
#9927=AXIS2_PLACEMENT_3D ( 'NONE', #6199, #13619, #11926 ) ;
#9946=VECTOR ( 'NONE', #17419, 1000.000000000000000 ) ;
#9953=VERTEX_POINT ( 'NONE', #532 ) ;
#9961=ADVANCED_FACE ( 'NONE', ( #16247 ), #14840, .T. ) ;
#9964=FACE_OUTER_BOUND ( 'NONE', #10118, .T. ) ;
#9976=ORIENTED_EDGE ( 'NONE', *, *, #9291, .F. ) ;
#9978=CARTESIAN_POINT ( 'NONE',  ( -66.71217848887407342, 56.48326379586188750, -24.23239327750837191 ) ) ;
#9989=FACE_OUTER_BOUND ( 'NONE', #3672, .T. ) ;
#9992=CARTESIAN_POINT ( 'NONE',  ( -12.80512717543878942, 28.43086510689403568, 39.77885264312817526 ) ) ;
#9999=CONICAL_SURFACE ( 'NONE', #4003, 3.999999999999989786, 1.029744258676652091 ) ;
#10004=ORIENTED_EDGE ( 'NONE', *, *, #8733, .T. ) ;
#10006=ADVANCED_FACE ( 'NONE', ( #15483 ), #15395, .F. ) ;
#10007=EDGE_LOOP ( 'NONE', ( #9433, #1858, #2429, #1368, #10464, #5099 ) ) ;
#10008=FACE_OUTER_BOUND ( 'NONE', #5288, .T. ) ;
#10011=CARTESIAN_POINT ( 'NONE',  ( -67.36180031798897971, 111.7399260588586287, -22.93227665730716325 ) ) ;
#10012=SHAPE_REPRESENTATION_RELATIONSHIP ( 'NONE' , 'NONE' ,  #17553, #7459 ) ;
#10015=VECTOR ( 'NONE', #10629, 1000.000000000000000 ) ;
#10030=CIRCLE ( 'NONE', #3414, 20.99999999999999645 ) ;
#10040=CARTESIAN_POINT ( 'NONE',  ( -68.12361985383350316, 84.22855780814606419, -28.00000000000000355 ) ) ;
#10043=CARTESIAN_POINT ( 'NONE',  ( -67.59262256747315689, 50.58224449241410525, 15.00000000000006750 ) ) ;
#10048=DIRECTION ( 'NONE',  ( -1.000000000000000000, -0.000000000000000000, -0.000000000000000000 ) ) ;
#10061=EDGE_LOOP ( 'NONE', ( #6316, #13462, #11586, #11189 ) ) ;
#10064=CARTESIAN_POINT ( 'NONE',  ( -127.5926225674731995, 110.5691553257988460, 30.35917033480641081 ) ) ;
#10068=PLANE ( 'NONE',  #3698 ) ;
#10075=EDGE_CURVE ( 'NONE', #13404, #10351, #18481, .T. ) ;
#10081=DIRECTION ( 'NONE',  ( -0.3197242186372270534, 0.9475106458593564041, 0.000000000000000000 ) ) ;
#10083=CARTESIAN_POINT ( 'NONE',  ( 15.23320273812467462, -111.0842361345572158, -3.000000000000000000 ) ) ;
#10087=EDGE_CURVE ( 'NONE', #10621, #14872, #16883, .T. ) ;
#10094=CARTESIAN_POINT ( 'NONE',  ( -92.59262256747321373, 117.8748711238780373, -15.00000000000000711 ) ) ;
#10095=CARTESIAN_POINT ( 'NONE',  ( -64.09025127992788384, 50.58224449241410525, 35.00000000000000000 ) ) ;
#10098=DIRECTION ( 'NONE',  ( -0.9475106458593564041, 0.3197242186372270534, 0.000000000000000000 ) ) ;
#10101=CARTESIAN_POINT ( 'NONE',  ( -40.53769224766538315, 54.09612659366786147, 24.44902958348917466 ) ) ;
#10104=EDGE_CURVE ( 'NONE', #6695, #15813, #11728, .T. ) ;
#10111=ORIENTED_EDGE ( 'NONE', *, *, #13726, .T. ) ;
#10115=DIRECTION ( 'NONE',  ( 4.675871521838984962E-16, -1.000000000000000000, 0.000000000000000000 ) ) ;
#10118=EDGE_LOOP ( 'NONE', ( #7573, #11603, #14732, #4160 ) ) ;
#10123=CONICAL_SURFACE ( 'NONE', #4432, 3.999999999999982681, 1.029744258676651203 ) ;
#10124=ORIENTED_EDGE ( 'NONE', *, *, #229, .T. ) ;
#10132=CARTESIAN_POINT ( 'NONE',  ( -83.12361985383351737, 84.22855780814606419, 37.50000000000000000 ) ) ;
#10150=CARTESIAN_POINT ( 'NONE',  ( 124.5381772159375942, -46.83756720124470263, -57.00000000000000000 ) ) ;
#10158=AXIS2_PLACEMENT_3D ( 'NONE', #2879, #7964, #12094 ) ;
#10163=CARTESIAN_POINT ( 'NONE',  ( -112.5926225674731995, 50.58224449241410525, 35.00000000000000000 ) ) ;
#10168=EDGE_CURVE ( 'NONE', #5660, #6083, #3130, .T. ) ;
#10172=CARTESIAN_POINT ( 'NONE',  ( -66.51364668169603078, 112.0410723289543995, -28.00000000000000355 ) ) ;
#10176=VERTEX_POINT ( 'NONE', #4778 ) ;
#10182=LINE ( 'NONE', #2816, #13911 ) ;
#10187=CIRCLE ( 'NONE', #9294, 20.99999999999999645 ) ;
#10190=EDGE_CURVE ( 'NONE', #11788, #18251, #4845, .T. ) ;
#10201=PLANE ( 'NONE',  #10901 ) ;
#10204=ADVANCED_FACE ( 'NONE', ( #11828 ), #1900, .F. ) ;
#10215=VECTOR ( 'NONE', #11537, 1000.000000000000000 ) ;
#10217=ORIENTED_EDGE ( 'NONE', *, *, #12500, .T. ) ;
#10219=B_SPLINE_CURVE_WITH_KNOTS ( 'NONE', 3,
 ( #16474, #2080, #17512, #10407, #16096, #10602 ),
 .UNSPECIFIED., .F., .F.,
 ( 4, 2, 4 ),
 ( 0.007841539089391896464, 0.008626660956717931844, 0.009411782824043968959 ),
 .UNSPECIFIED. ) ;
#10221=CARTESIAN_POINT ( 'NONE',  ( -64.09025127992791226, 117.8748711238780373, 35.00000000000000000 ) ) ;
#10229=CARTESIAN_POINT ( 'NONE',  ( -123.4618227840623632, -111.0842361345572158, 57.00000000000000000 ) ) ;
#10235=EDGE_LOOP ( 'NONE', ( #1611, #15089, #2319, #8672 ) ) ;
#10239=ORIENTED_EDGE ( 'NONE', *, *, #14454, .F. ) ;
#10241=CARTESIAN_POINT ( 'NONE',  ( -67.59262256747317110, 61.64996188551982215, 25.00000000000000355 ) ) ;
#10251=CIRCLE ( 'NONE', #10539, 11.04359719766049430 ) ;
#10252=VECTOR ( 'NONE', #384, 1000.000000000000000 ) ;
#10255=CARTESIAN_POINT ( 'NONE',  ( -70.06856178257687873, 57.88796029049330372, 22.35917033480642502 ) ) ;
#10260=EDGE_LOOP ( 'NONE', ( #9453, #16121, #16986, #10889, #12736, #16620, #9568, #1363, #5916, #18078, #12569, #15872 ) ) ;
#10263=VECTOR ( 'NONE', #17854, 1000.000000000000000 ) ;
#10266=DIRECTION ( 'NONE',  ( 1.000000000000000000, -0.000000000000000000, -0.000000000000000000 ) ) ;
#10269=CARTESIAN_POINT ( 'NONE',  ( -67.59262256747317110, 57.88796029049329661, -26.35917033480641436 ) ) ;
#10273=AXIS2_PLACEMENT_3D ( 'NONE', #6012, #12981, #1646 ) ;
#10281=VECTOR ( 'NONE', #4245, 1000.000000000000114 ) ;
#10295=FACE_OUTER_BOUND ( 'NONE', #18056, .T. ) ;
#10299=CARTESIAN_POINT ( 'NONE',  ( -127.5926225674731995, 110.5691553257988460, 26.35917033480641436 ) ) ;
#10313=CIRCLE ( 'NONE', #5226, 18.23991632971910803 ) ;
#10317=EDGE_CURVE ( 'NONE', #9318, #8476, #3669, .T. ) ;
#10320=ORIENTED_EDGE ( 'NONE', *, *, #14526, .F. ) ;
#10351=VERTEX_POINT ( 'NONE', #8350 ) ;
#10362=FACE_OUTER_BOUND ( 'NONE', #1190, .T. ) ;
#10364=CARTESIAN_POINT ( 'NONE',  ( 15.23320273812466041, 0.000000000000000000, -3.000000000000000000 ) ) ;
#10365=ORIENTED_EDGE ( 'NONE', *, *, #14546, .T. ) ;
#10367=DIRECTION ( 'NONE',  ( 1.000000000000000000, 0.000000000000000000, 0.000000000000000000 ) ) ;
#10377=ORIENTED_EDGE ( 'NONE', *, *, #14438, .F. ) ;
#10379=CARTESIAN_POINT ( 'NONE',  ( 9.543663295069050534, 56.41207303426870112, 7.000000000000010658 ) ) ;
#10382=DIRECTION ( 'NONE',  ( 0.000000000000000000, 0.000000000000000000, 1.000000000000000000 ) ) ;
#10387=ADVANCED_FACE ( 'NONE', ( #2739 ), #9561, .T. ) ;
#10399=LINE ( 'NONE', #10221, #15971 ) ;
#10407=CARTESIAN_POINT ( 'NONE',  ( -66.05502429040123502, 111.0949457325500163, 25.00000000000000355 ) ) ;
#10409=EDGE_CURVE ( 'NONE', #4575, #6976, #394, .T. ) ;
#10413=DIRECTION ( 'NONE',  ( -0.000000000000000000, -0.000000000000000000, -1.000000000000000000 ) ) ;
#10414=ORIENTED_EDGE ( 'NONE', *, *, #5149, .T. ) ;
#10423=DIRECTION ( 'NONE',  ( -1.000000000000000000, 0.000000000000000000, 0.000000000000000000 ) ) ;
#10432=FACE_OUTER_BOUND ( 'NONE', #5931, .T. ) ;
#10441=VECTOR ( 'NONE', #11475, 1000.000000000000000 ) ;
#10447=CARTESIAN_POINT ( 'NONE',  ( -31.03642545851250745, 84.22855780814606419, 37.50000000000000000 ) ) ;
#10460=DIRECTION ( 'NONE',  ( -0.000000000000000000, 1.200240087506842815E-16, 1.000000000000000000 ) ) ;
#10464=ORIENTED_EDGE ( 'NONE', *, *, #15322, .T. ) ;
#10469=CARTESIAN_POINT ( 'NONE',  ( -64.09025127992788384, 50.58224449241409104, -35.00000000000000000 ) ) ;
#10486=CARTESIAN_POINT ( 'NONE',  ( -67.59262256747319952, 111.6514400295689171, 22.50837044127971254 ) ) ;
#10487=CARTESIAN_POINT ( 'NONE',  ( -57.08002265617300708, 84.22855780814606419, -28.00000000000000355 ) ) ;
#10497=VECTOR ( 'NONE', #12, 1000.000000000000000 ) ;
#10501=ORIENTED_EDGE ( 'NONE', *, *, #1405, .T. ) ;
#10510=CIRCLE ( 'NONE', #14415, 20.99999999999998934 ) ;
#10513=ORIENTED_EDGE ( 'NONE', *, *, #3208, .F. ) ;
#10522=DIRECTION ( 'NONE',  ( 1.000000000000000000, 2.062304371594500494E-16, -0.000000000000000000 ) ) ;
#10527=PLANE ( 'NONE',  #14766 ) ;
#10530=VERTEX_POINT ( 'NONE', #10040 ) ;
#10531=VERTEX_POINT ( 'NONE', #2927 ) ;
#10532=EDGE_CURVE ( 'NONE', #8271, #2272, #14684, .T. ) ;
#10539=AXIS2_PLACEMENT_3D ( 'NONE', #14772, #17663, #1966 ) ;
#10545=LINE ( 'NONE', #183, #5463 ) ;
#10554=VECTOR ( 'NONE', #2391, 1000.000000000000000 ) ;
#10556=DIRECTION ( 'NONE',  ( 0.000000000000000000, 0.000000000000000000, 1.000000000000000000 ) ) ;
#10562=VECTOR ( 'NONE', #13891, 1000.000000000000000 ) ;
#10564=DIRECTION ( 'NONE',  ( -0.000000000000000000, 0.000000000000000000, -1.000000000000000000 ) ) ;
#10565=ORIENTED_EDGE ( 'NONE', *, *, #17478, .F. ) ;
#10568=CARTESIAN_POINT ( 'NONE',  ( -72.32324610293285616, 109.3399659331339677, 22.53855496370561440 ) ) ;
#10570=CIRCLE ( 'NONE', #13564, 11.04359719766049430 ) ;
#10575=ORIENTED_EDGE ( 'NONE', *, *, #2983, .T. ) ;
#10578=CARTESIAN_POINT ( 'NONE',  ( -76.14195937732675645, 61.88640485328121343, -26.51881048504861482 ) ) ;
#10579=CARTESIAN_POINT ( 'NONE',  ( -67.59262256747317110, 57.88796029049329661, -30.35917033480639660 ) ) ;
#10588=CIRCLE ( 'NONE', #9402, 180.8515291679561585 ) ;
#10601=DIRECTION ( 'NONE',  ( -1.000000000000000000, 0.000000000000000000, 0.000000000000000000 ) ) ;
#10602=CARTESIAN_POINT ( 'NONE',  ( -66.00585202009862940, 110.5691553257988460, 25.00000000000000355 ) ) ;
#10606=CIRCLE ( 'NONE', #11204, 26.04359719766049608 ) ;
#10608=ORIENTED_EDGE ( 'NONE', *, *, #14853, .F. ) ;
#10621=VERTEX_POINT ( 'NONE', #14430 ) ;
#10628=VECTOR ( 'NONE', #14748, 1000.000000000000000 ) ;
#10629=DIRECTION ( 'NONE',  ( -0.000000000000000000, -0.000000000000000000, 1.000000000000000000 ) ) ;
#10632=VERTEX_POINT ( 'NONE', #14517 ) ;
#10636=ADVANCED_FACE ( 'NONE', ( #17573 ), #4755, .F. ) ;
#10639=ADVANCED_FACE ( 'NONE', ( #16450 ), #17951, .F. ) ;
#10640=ORIENTED_EDGE ( 'NONE', *, *, #11657, .F. ) ;
#10645=CARTESIAN_POINT ( 'NONE',  ( -102.4618227840623774, -111.0842361345572158, -36.00000000000000000 ) ) ;
#10650=EDGE_CURVE ( 'NONE', #3501, #18444, #9356, .T. ) ;
#10667=CARTESIAN_POINT ( 'NONE',  ( -73.62694592582826658, 108.4942417827056289, 22.93390062366417936 ) ) ;
#10670=FACE_OUTER_BOUND ( 'NONE', #6416, .T. ) ;
#10677=ORIENTED_EDGE ( 'NONE', *, *, #8239, .F. ) ;
#10684=ORIENTED_EDGE ( 'NONE', *, *, #16942, .T. ) ;
#10694=EDGE_CURVE ( 'NONE', #14649, #18482, #18452, .T. ) ;
#10702=CARTESIAN_POINT ( 'NONE',  ( -100.4870060002411805, -151.5628872026273086, 18.23991632971911869 ) ) ;
#10721=VECTOR ( 'NONE', #10115, 1000.000000000000000 ) ;
#10729=CARTESIAN_POINT ( 'NONE',  ( 105.4583593777967963, -32.62665103886256190, -7.000000000000010658 ) ) ;
#10745=CARTESIAN_POINT ( 'NONE',  ( -71.20513298132846103, 58.47161403914679312, 22.38837701002785607 ) ) ;
#10748=DIRECTION ( 'NONE',  ( -0.000000000000000000, -0.000000000000000000, 1.000000000000000000 ) ) ;
#10751=VECTOR ( 'NONE', #18374, 1000.000000000000000 ) ;
#10753=DIRECTION ( 'NONE',  ( 0.000000000000000000, 0.000000000000000000, -1.000000000000000000 ) ) ;
#10755=DIRECTION ( 'NONE',  ( -0.000000000000000000, -0.000000000000000000, 1.000000000000000000 ) ) ;
#10771=CARTESIAN_POINT ( 'NONE',  ( -42.22262702428728431, 53.23066522635949838, -25.06792223060221048 ) ) ;
#10779=CARTESIAN_POINT ( 'NONE',  ( -57.08002265617300708, 84.22855780814606419, 7.000000000000009770 ) ) ;
#10780=AXIS2_PLACEMENT_3D ( 'NONE', #2582, #15102, #5359 ) ;
#10793=FACE_OUTER_BOUND ( 'NONE', #5438, .T. ) ;
#10805=DIRECTION ( 'NONE',  ( 0.000000000000000000, 0.000000000000000000, 1.000000000000000000 ) ) ;
#10808=LINE ( 'NONE', #3793, #16739 ) ;
#10824=CIRCLE ( 'NONE', #3335, 3.999999999999989786 ) ;
#10851=VECTOR ( 'NONE', #5804, 1000.000000000000000 ) ;
#10854=DIRECTION ( 'NONE',  ( 0.000000000000000000, -0.000000000000000000, 1.000000000000000000 ) ) ;
#10860=ORIENTED_EDGE ( 'NONE', *, *, #14075, .F. ) ;
#10863=EDGE_CURVE ( 'NONE', #8038, #1895, #5472, .T. ) ;
#10864=CIRCLE ( 'NONE', #15346, 29.36884788726140627 ) ;
#10865=CARTESIAN_POINT ( 'NONE',  ( -194.4437806548868934, -111.0842361345572158, -18.23991632971910803 ) ) ;
#10868=CARTESIAN_POINT ( 'NONE',  ( -70.71978124295696944, -141.5628872026273086, -18.23991632971910803 ) ) ;
#10869=DIRECTION ( 'NONE',  ( -0.000000000000000000, 0.000000000000000000, 1.000000000000000000 ) ) ;
#10880=DIRECTION ( 'NONE',  ( -0.000000000000000000, 1.000000000000000000, -0.000000000000000000 ) ) ;
#10882=B_SPLINE_CURVE_WITH_KNOTS ( 'NONE', 3,
 ( #6899, #1200, #4099, #5492, #12625, #9802, #7668, #4953, #10667, #11703, #10568, #17664, #378, #16164, #16352, #16271 ),
 .UNSPECIFIED., .F., .F.,
 ( 4, 2, 2, 2, 2, 2, 2, 4 ),
 ( 0.000000000000000000, 0.0009642797493039184610, 0.001928559498607836922, 0.002892839247911755708, 0.003857118997215673844, 0.005785678495823502743, 0.006749958245127435190, 0.007714237994431366770 ),
 .UNSPECIFIED. ) ;
#10889=ORIENTED_EDGE ( 'NONE', *, *, #14853, .T. ) ;
#10891=EDGE_CURVE ( 'NONE', #4298, #2330, #12795, .T. ) ;
#10901=AXIS2_PLACEMENT_3D ( 'NONE', #5708, #14328, #7310 ) ;
#10910=CARTESIAN_POINT ( 'NONE',  ( -76.04905332431492582, 106.6498183473933068, -27.18785666068412610 ) ) ;
#10911=CARTESIAN_POINT ( 'NONE',  ( -66.00585202009862940, 110.5691553257988460, 25.00000000000000355 ) ) ;
#10912=ORIENTED_EDGE ( 'NONE', *, *, #7545, .F. ) ;
#10919=B_SPLINE_CURVE_WITH_KNOTS ( 'NONE', 3,
 ( #13188, #7468, #3253, #271, #11781, #7658, #14668, #367, #3175, #11954, #4568, #6230 ),
 .UNSPECIFIED., .F., .F.,
 ( 4, 2, 2, 2, 2, 4 ),
 ( 0.01258489339592914341, 0.01361446459519792193, 0.01464403579446670045, 0.01567360699373548244, 0.01618839259336985956, 0.01670317819300424014 ),
 .UNSPECIFIED. ) ;
#10923=EDGE_CURVE ( 'NONE', #3472, #13404, #1905, .T. ) ;
#10927=CARTESIAN_POINT ( 'NONE',  ( 105.4583593777967963, -32.62665103886256190, 7.000000000000010658 ) ) ;
#10929=VERTEX_POINT ( 'NONE', #5380 ) ;
#10949=CARTESIAN_POINT ( 'NONE',  ( -66.17295708481962890, 57.85212116841895380, -28.00000000000000355 ) ) ;
#10950=CARTESIAN_POINT ( 'NONE',  ( -44.49764538373973721, 84.22855780814606419, 37.50000000000000000 ) ) ;
#10955=PLANE ( 'NONE',  #15250 ) ;
#10965=FACE_OUTER_BOUND ( 'NONE', #11414, .T. ) ;
#10970=ORIENTED_EDGE ( 'NONE', *, *, #10409, .T. ) ;
#10983=FACE_OUTER_BOUND ( 'NONE', #10061, .T. ) ;
#10990=DIRECTION ( 'NONE',  ( 0.000000000000000000, 0.000000000000000000, -1.000000000000000000 ) ) ;
#10991=VERTEX_POINT ( 'NONE', #8200 ) ;
#10994=DIRECTION ( 'NONE',  ( 1.119176436114069332E-16, -1.000000000000000000, -0.000000000000000000 ) ) ;
#10996=CARTESIAN_POINT ( 'NONE',  ( -67.59262256747319952, 110.5691553257988460, 30.35917033480640370 ) ) ;
#11002=CARTESIAN_POINT ( 'NONE',  ( -67.59262256747317110, 56.80567558672318995, -22.50837044127973030 ) ) ;
#11007=ORIENTED_EDGE ( 'NONE', *, *, #11233, .F. ) ;
#11008=ORIENTED_EDGE ( 'NONE', *, *, #2524, .T. ) ;
#11013=CYLINDRICAL_SURFACE ( 'NONE', #17053, 34.36884788726141693 ) ;
#11015=DIRECTION ( 'NONE',  ( -1.000000000000000000, 0.000000000000000000, 0.000000000000000000 ) ) ;
#11020=LINE ( 'NONE', #906, #2870 ) ;
#11035=CARTESIAN_POINT ( 'NONE',  ( -66.01768795098074349, 57.62469735380677349, 25.00000000000000355 ) ) ;
#11045=ORIENTED_EDGE ( 'NONE', *, *, #17723, .F. ) ;
#11048=CARTESIAN_POINT ( 'NONE',  ( -69.26154997389620860, 57.49002305898234511, 22.35917033480642502 ) ) ;
#11056=DIRECTION ( 'NONE',  ( 1.000000000000000000, 0.000000000000000000, 0.000000000000000000 ) ) ;
#11063=LINE ( 'NONE', #1069, #4524 ) ;
#11068=CARTESIAN_POINT ( 'NONE',  ( -127.5926225674731995, 106.9211863004614997, -28.00000000000000355 ) ) ;
#11070=VECTOR ( 'NONE', #5697, 1000.000000000000000 ) ;
#11072=AXIS2_PLACEMENT_3D ( 'NONE', #14120, #11405, #15426 ) ;
#11079=AXIS2_PLACEMENT_3D ( 'NONE', #14142, #10460, #7659 ) ;
#11085=CARTESIAN_POINT ( 'NONE',  ( -64.09025127992789805, 84.22855780814606419, 28.00000000000000355 ) ) ;
#11092=CARTESIAN_POINT ( 'NONE',  ( -127.5926225674731995, 117.8748711238780373, -15.00000000000000355 ) ) ;
#11095=EDGE_CURVE ( 'NONE', #10929, #535, #3044, .T. ) ;
#11097=EDGE_CURVE ( 'NONE', #8646, #15955, #4624, .T. ) ;
#11101=AXIS2_PLACEMENT_3D ( 'NONE', #1267, #18000, #14180 ) ;
#11129=PLANE ( 'NONE',  #14938 ) ;
#11130=ORIENTED_EDGE ( 'NONE', *, *, #3097, .F. ) ;
#11137=CARTESIAN_POINT ( 'NONE',  ( -74.36154358637296014, 60.48060622302846667, 23.30558296767449278 ) ) ;
#11138=CARTESIAN_POINT ( 'NONE',  ( -66.00585202009861518, 57.75741913890266943, 25.00000000000001066 ) ) ;
#11143=ORIENTED_EDGE ( 'NONE', *, *, #6412, .F. ) ;
#11146=CARTESIAN_POINT ( 'NONE',  ( -70.85175816390371040, -141.5628872026273086, -57.00000000000000000 ) ) ;
#11159=DIRECTION ( 'NONE',  ( 0.000000000000000000, 1.000000000000000000, 0.000000000000000000 ) ) ;
#11167=EDGE_LOOP ( 'NONE', ( #17865, #8185, #8173, #2973 ) ) ;
#11171=CARTESIAN_POINT ( 'NONE',  ( -67.59262256747317110, 57.88796029049329661, 26.35917033480641436 ) ) ;
#11172=EDGE_LOOP ( 'NONE', ( #11547, #2961 ) ) ;
#11176=EDGE_CURVE ( 'NONE', #11585, #6695, #1724, .T. ) ;
#11177=VERTEX_POINT ( 'NONE', #13238 ) ;
#11185=CARTESIAN_POINT ( 'NONE',  ( 95.45835937779683888, -32.62665103886254059, -7.000000000000010658 ) ) ;
#11189=ORIENTED_EDGE ( 'NONE', *, *, #931, .F. ) ;
#11191=VECTOR ( 'NONE', #3070, 1000.000000000000000 ) ;
#11193=DIRECTION ( 'NONE',  ( 1.000000000000000000, 0.000000000000000000, 0.000000000000000000 ) ) ;
#11194=CARTESIAN_POINT ( 'NONE',  ( -66.51364668169603078, 112.0410723289543995, -28.00000000000000355 ) ) ;
#11196=B_SPLINE_CURVE_WITH_KNOTS ( 'NONE', 3,
 ( #15537, #8338, #15645, #2729 ),
 .UNSPECIFIED., .F., .F.,
 ( 4, 4 ),
 ( 0.01093108579351914633, 0.01364771765276243456 ),
 .UNSPECIFIED. ) ;
#11199=CARTESIAN_POINT ( 'NONE',  ( -66.17203968311494577, 56.30249863064624094, -26.82861026404109239 ) ) ;
#11204=AXIS2_PLACEMENT_3D ( 'NONE', #13959, #1141, #18258 ) ;
#11209=DIRECTION ( 'NONE',  ( -1.156482317317869999E-16, 0.000000000000000000, -1.000000000000000000 ) ) ;
#11215=EDGE_CURVE ( 'NONE', #4466, #2953, #1124, .T. ) ;
#11219=CARTESIAN_POINT ( 'NONE',  ( -10.92059662857647240, 26.05810099730991070, -40.87008517519171136 ) ) ;
#11224=VECTOR ( 'NONE', #4028, 1000.000000000000000 ) ;
#11227=LINE ( 'NONE', #6811, #898 ) ;
#11232=EDGE_LOOP ( 'NONE', ( #3856, #2956, #4985, #17799, #10239, #13288 ) ) ;
#11233=EDGE_CURVE ( 'NONE', #17254, #3060, #4037, .T. ) ;
#11234=FACE_BOUND ( 'NONE', #17686, .T. ) ;
#11238=CARTESIAN_POINT ( 'NONE',  ( -67.15841416737785607, 56.64230282782159520, 23.31749251357070918 ) ) ;
#11239=CARTESIAN_POINT ( 'NONE',  ( -123.4618227840623632, -111.0842361345572158, -18.23991632971910803 ) ) ;
#11241=ORIENTED_EDGE ( 'NONE', *, *, #10104, .F. ) ;
#11244=CARTESIAN_POINT ( 'NONE',  ( -66.47936379154189979, 109.1731751823756014, -28.00000000000000000 ) ) ;
#11247=CARTESIAN_POINT ( 'NONE',  ( 9.543663295069050534, 56.41207303426870112, 3.000000000000000000 ) ) ;
#11249=EDGE_CURVE ( 'NONE', #17198, #8524, #13940, .T. ) ;
#11265=EDGE_CURVE ( 'NONE', #15284, #16629, #14936, .T. ) ;
#11270=B_SPLINE_CURVE_WITH_KNOTS ( 'NONE', 3,
 ( #9228, #726, #6418, #2212, #12141, #16416, #7925, #12220, #17916, #16517, #3715, #9425, #15120, #13716, #18314, #9893, #63, #9992, #6800, #16902, #15700, #11395, #18217, #9796, #2497, #15601 ),
 .UNSPECIFIED., .F., .F.,
 ( 4, 2, 2, 2, 2, 2, 2, 2, 2, 2, 2, 2, 4 ),
 ( 6.992893892674702526E-18, 0.01247275093652063134, 0.01870912640478094788, 0.02182731413891110528, 0.02494550187304126268, 0.03741825280956187494, 0.04365462827782218974, 0.04677281601195235755, 0.04989100374608251842, 0.06236375468260317578, 0.07483650561912381927, 0.08730925655564447663, 0.09978200749216512011 ),
 .UNSPECIFIED. ) ;
#11284=CARTESIAN_POINT ( 'NONE',  ( -64.09025127992791226, 109.3109350805793270, 28.00000000000000355 ) ) ;
#11287=VERTEX_POINT ( 'NONE', #12453 ) ;
#11288=DIRECTION ( 'NONE',  ( -0.000000000000000000, -0.000000000000000000, 1.000000000000000000 ) ) ;
#11295=CARTESIAN_POINT ( 'NONE',  ( -67.13578943540532862, 56.63396920285576641, -23.36002886201060846 ) ) ;
#11296=ORIENTED_EDGE ( 'NONE', *, *, #8452, .T. ) ;
#11307=CARTESIAN_POINT ( 'NONE',  ( -34.76410658286479816, 45.09554562204261430, -30.51224260568122304 ) ) ;
#11314=EDGE_LOOP ( 'NONE', ( #7864, #17434 ) ) ;
#11318=ORIENTED_EDGE ( 'NONE', *, *, #13073, .T. ) ;
#11324=FACE_OUTER_BOUND ( 'NONE', #15660, .T. ) ;
#11325=CARTESIAN_POINT ( 'NONE',  ( -92.59262256747321373, 117.8748711238780373, 15.00000000000006040 ) ) ;
#11329=EDGE_CURVE ( 'NONE', #11975, #2362, #10570, .T. ) ;
#11334=ORIENTED_EDGE ( 'NONE', *, *, #2706, .F. ) ;
#11337=EDGE_CURVE ( 'NONE', #13685, #6726, #902, .T. ) ;
#11343=EDGE_CURVE ( 'NONE', #4543, #1922, #5503, .T. ) ;
#11350=ORIENTED_EDGE ( 'NONE', *, *, #8517, .F. ) ;
#11352=AXIS2_PLACEMENT_3D ( 'NONE', #10163, #176, #6204 ) ;
#11355=DIRECTION ( 'NONE',  ( -0.000000000000000000, -0.000000000000000000, -1.000000000000000000 ) ) ;
#11370=CARTESIAN_POINT ( 'NONE',  ( -12.34732335292710559, 42.05992578482485555, -32.40189210255460495 ) ) ;
#11380=ORIENTED_EDGE ( 'NONE', *, *, #14526, .T. ) ;
#11387=EDGE_LOOP ( 'NONE', ( #1959, #4546, #7389, #3449 ) ) ;
#11394=AXIS2_PLACEMENT_3D ( 'NONE', #4092, #11209, #6704 ) ;
#11395=CARTESIAN_POINT ( 'NONE',  ( -31.19111409321185846, 43.29857725109086175, 31.64380382776071343 ) ) ;
#11404=DIRECTION ( 'NONE',  ( 1.000000000000000000, 0.000000000000000000, 0.000000000000000000 ) ) ;
#11405=DIRECTION ( 'NONE',  ( 1.000000000000000000, 2.062304371594500494E-16, -0.000000000000000000 ) ) ;
#11414=EDGE_LOOP ( 'NONE', ( #9155, #16715, #16796, #3359, #11933 ) ) ;
#11415=CARTESIAN_POINT ( 'NONE',  ( -67.13594510831309492, 111.8230895504084117, -23.35973016812594949 ) ) ;
#11418=CARTESIAN_POINT ( 'NONE',  ( -66.18295968148926534, 110.2709693283236874, -28.00000000000000000 ) ) ;
#11429=VERTEX_POINT ( 'NONE', #5952 ) ;
#11434=EDGE_CURVE ( 'NONE', #13472, #14911, #2024, .T. ) ;
#11437=CARTESIAN_POINT ( 'NONE',  ( 95.45835937779679625, 56.41207303426869402, -7.000000000000010658 ) ) ;
#11440=CARTESIAN_POINT ( 'NONE',  ( -123.4618227840623632, -111.0842361345572158, -57.00000000000000000 ) ) ;
#11442=CARTESIAN_POINT ( 'NONE',  ( 124.5381772159375942, -111.0842361345572158, 7.000000000000010658 ) ) ;
#11475=DIRECTION ( 'NONE',  ( 0.000000000000000000, 0.000000000000000000, 1.000000000000000000 ) ) ;
#11479=ORIENTED_EDGE ( 'NONE', *, *, #3418, .T. ) ;
#11482=CARTESIAN_POINT ( 'NONE',  ( -67.59262256747319952, 110.5691553257988460, -26.35917033480641436 ) ) ;
#11503=CARTESIAN_POINT ( 'NONE',  ( 15.23320273812466041, -19.34983604512934363, -54.79921157549233612 ) ) ;
#11504=VERTEX_POINT ( 'NONE', #3331 ) ;
#11513=CARTESIAN_POINT ( 'NONE',  ( -67.59262256747319952, 111.6514400295689171, -22.50837044127971254 ) ) ;
#11518=DIRECTION ( 'NONE',  ( -0.000000000000000000, -0.000000000000000000, 1.000000000000000000 ) ) ;
#11524=ORIENTED_EDGE ( 'NONE', *, *, #15900, .F. ) ;
#11525=EDGE_CURVE ( 'NONE', #4466, #10176, #1939, .T. ) ;
#11537=DIRECTION ( 'NONE',  ( 2.062304371594500494E-16, -1.000000000000000000, 1.073258342404370555E-31 ) ) ;
#11543=VECTOR ( 'NONE', #7029, 1000.000000000000000 ) ;
#11547=ORIENTED_EDGE ( 'NONE', *, *, #8934, .T. ) ;
#11548=EDGE_CURVE ( 'NONE', #3566, #13829, #15676, .T. ) ;
#11549=DIRECTION ( 'NONE',  ( 0.000000000000000000, 0.000000000000000000, -1.000000000000000000 ) ) ;
#11556=DIRECTION ( 'NONE',  ( -1.000000000000000000, -0.000000000000000000, -0.000000000000000000 ) ) ;
#11566=EDGE_CURVE ( 'NONE', #14497, #1479, #1914, .T. ) ;
#11583=ADVANCED_FACE ( 'NONE', ( #8205 ), #5204, .F. ) ;
#11584=LINE ( 'NONE', #433, #17632 ) ;
#11585=VERTEX_POINT ( 'NONE', #13817 ) ;
#11586=ORIENTED_EDGE ( 'NONE', *, *, #10863, .F. ) ;
#11588=CARTESIAN_POINT ( 'NONE',  ( 15.23320273812466041, -46.83756720124470263, -115.7605492041889619 ) ) ;
#11590=CARTESIAN_POINT ( 'NONE',  ( -66.28651633149024747, 112.1171927384383764, -25.37060304889219609 ) ) ;
#11591=DIRECTION ( 'NONE',  ( -0.000000000000000000, -0.000000000000000000, -1.000000000000000000 ) ) ;
#11603=ORIENTED_EDGE ( 'NONE', *, *, #8009, .F. ) ;
#11609=CARTESIAN_POINT ( 'NONE',  ( -123.4618227840623632, -151.5628872026273086, 57.00000000000000000 ) ) ;
#11624=LINE ( 'NONE', #8560, #17438 ) ;
#11641=ADVANCED_FACE ( 'NONE', ( #2213 ), #8098, .F. ) ;
#11646=DIRECTION ( 'NONE',  ( -0.000000000000000000, -0.000000000000000000, 1.000000000000000000 ) ) ;
#11649=LINE ( 'NONE', #8940, #18065 ) ;
#11657=EDGE_CURVE ( 'NONE', #15955, #16713, #7594, .T. ) ;
#11688=LINE ( 'NONE', #6049, #6578 ) ;
#11696=VECTOR ( 'NONE', #6582, 1000.000000000000000 ) ;
#11703=CARTESIAN_POINT ( 'NONE',  ( -72.85813335477966746, 109.0067719868844449, 22.65648029595582358 ) ) ;
#11704=CYLINDRICAL_SURFACE ( 'NONE', #12876, 3.999999999999996447 ) ;
#11707=CARTESIAN_POINT ( 'NONE',  ( -127.5926225674732279, 47.87487112387803023, 15.00000000000004263 ) ) ;
#11715=CARTESIAN_POINT ( 'NONE',  ( -57.08002265617300708, 84.22855780814606419, -28.00000000000000355 ) ) ;
#11728=LINE ( 'NONE', #17244, #9946 ) ;
#11729=ORIENTED_EDGE ( 'NONE', *, *, #5047, .F. ) ;
#11734=ORIENTED_EDGE ( 'NONE', *, *, #468, .T. ) ;
#11741=CARTESIAN_POINT ( 'NONE',  ( -123.4618227840623632, -111.0842361345572158, -7.000000000000013323 ) ) ;
#11744=CARTESIAN_POINT ( 'NONE',  ( -57.08002265617300708, 84.22855780814606419, 37.50000000000000000 ) ) ;
#11748=CARTESIAN_POINT ( 'NONE',  ( -100.4870060002411805, -151.5628872026273086, -57.00000000000000000 ) ) ;
#11760=VECTOR ( 'NONE', #2595, 1000.000000000000000 ) ;
#11766=CARTESIAN_POINT ( 'NONE',  ( -66.14901650176582848, 112.1621247781131530, -26.09456109111725652 ) ) ;
#11781=CARTESIAN_POINT ( 'NONE',  ( -66.76897068454591988, 60.14546051432880347, 25.00000000000000355 ) ) ;
#11788=VERTEX_POINT ( 'NONE', #16038 ) ;
#11791=EDGE_CURVE ( 'NONE', #15813, #1951, #16253, .T. ) ;
#11794=DIRECTION ( 'NONE',  ( -1.000000000000000000, 0.000000000000000000, 0.000000000000000000 ) ) ;
#11800=CARTESIAN_POINT ( 'NONE',  ( -92.59262256747321373, 117.8748711238780373, 15.00000000000005862 ) ) ;
#11811=DIRECTION ( 'NONE',  ( -0.000000000000000000, -0.000000000000000000, 1.000000000000000000 ) ) ;
#11817=EDGE_CURVE ( 'NONE', #16505, #1922, #11649, .T. ) ;
#11822=STYLED_ITEM('',(#18538),#12831);
#11828=FACE_OUTER_BOUND ( 'NONE', #12424, .T. ) ;
#11831=ORIENTED_EDGE ( 'NONE', *, *, #15560, .T. ) ;
#11834=ORIENTED_EDGE ( 'NONE', *, *, #12840, .F. ) ;
#11841=DIRECTION ( 'NONE',  ( -0.000000000000000000, -0.000000000000000000, 1.000000000000000000 ) ) ;
#11843=LINE ( 'NONE', #5769, #14991 ) ;
#11844=ORIENTED_EDGE ( 'NONE', *, *, #14508, .T. ) ;
#11856=VERTEX_POINT ( 'NONE', #325 ) ;
#11871=CARTESIAN_POINT ( 'NONE',  ( -127.5926225674731995, 110.5691553257988460, -26.35917033480641436 ) ) ;
#11880=CARTESIAN_POINT ( 'NONE',  ( -50.06979403241810900, 50.58224449241409104, -26.91246033477409583 ) ) ;
#11888=ORIENTED_EDGE ( 'NONE', *, *, #9835, .F. ) ;
#11894=CARTESIAN_POINT ( 'NONE',  ( 9.543663295069050534, 56.41207303426870112, -7.000000000000010658 ) ) ;
#11896=EDGE_LOOP ( 'NONE', ( #12925, #225, #2765, #6003, #17084, #5350, #15891, #4988, #15582, #7077 ) ) ;
#11900=ORIENTED_EDGE ( 'NONE', *, *, #2908, .F. ) ;
#11916=FACE_OUTER_BOUND ( 'NONE', #15846, .T. ) ;
#11917=DIRECTION ( 'NONE',  ( 1.000000000000000000, 0.000000000000000000, 0.000000000000000000 ) ) ;
#11920=EDGE_CURVE ( 'NONE', #7572, #6830, #8806, .T. ) ;
#11926=DIRECTION ( 'NONE',  ( -1.000000000000000000, 0.000000000000000000, 0.000000000000000000 ) ) ;
#11927=CARTESIAN_POINT ( 'NONE',  ( -92.59262256747321373, 117.8748711238780373, 35.00000000000000000 ) ) ;
#11929=VECTOR ( 'NONE', #18425, 1000.000000000000000 ) ;
#11933=ORIENTED_EDGE ( 'NONE', *, *, #687, .T. ) ;
#11939=CONICAL_SURFACE ( 'NONE', #10158, 3.999999999999982681, 1.029744258676651203 ) ;
#11949=CARTESIAN_POINT ( 'NONE',  ( 113.3630170098442989, -111.0842361345572158, 7.000000000000010658 ) ) ;
#11950=EDGE_LOOP ( 'NONE', ( #6481, #12850, #13060, #2841 ) ) ;
#11954=CARTESIAN_POINT ( 'NONE',  ( -66.02602711314098372, 58.23015000473216674, 25.00000000000000355 ) ) ;
#11962=DIRECTION ( 'NONE',  ( 0.000000000000000000, 0.000000000000000000, 1.000000000000000000 ) ) ;
#11975=VERTEX_POINT ( 'NONE', #13418 ) ;
#11984=CARTESIAN_POINT ( 'NONE',  ( -127.5926225674731711, 57.88796029049329661, 26.35917033480641436 ) ) ;
#11990=ADVANCED_FACE ( 'NONE', ( #6683 ), #7983, .F. ) ;
#11994=DIRECTION ( 'NONE',  ( 0.000000000000000000, 1.000000000000000000, 0.000000000000000000 ) ) ;
#11995=CARTESIAN_POINT ( 'NONE',  ( -92.59262256747321373, 110.5691553257988460, -26.35917033480641436 ) ) ;
#11996=CARTESIAN_POINT ( 'NONE',  ( 0.000000000000000000, 0.000000000000000000, -3.000000000000000000 ) ) ;
#12002=ORIENTED_EDGE ( 'NONE', *, *, #2182, .F. ) ;
#12007=EDGE_CURVE ( 'NONE', #4073, #8650, #15283, .T. ) ;
#12009=VERTEX_POINT ( 'NONE', #10702 ) ;
#12013=CARTESIAN_POINT ( 'NONE',  ( -57.08002265617300708, 84.22855780814606419, 37.50000000000000000 ) ) ;
#12026=CARTESIAN_POINT ( 'NONE',  ( -67.59262256747317110, 57.88796029049329661, -26.35917033480641436 ) ) ;
#12029=AXIS2_PLACEMENT_3D ( 'NONE', #2029, #7733, #6322 ) ;
#12030=CARTESIAN_POINT ( 'NONE',  ( 95.45835937779679625, 56.41207303426869402, -3.000000000000000000 ) ) ;
#12034=EDGE_CURVE ( 'NONE', #3387, #9128, #17893, .T. ) ;
#12044=AXIS2_PLACEMENT_3D ( 'NONE', #16435, #10564, #17764 ) ;
#12045=CARTESIAN_POINT ( 'NONE',  ( -112.5926225674731995, 50.58224449241410525, -15.00000000000000000 ) ) ;
#12049=CARTESIAN_POINT ( 'NONE',  ( -70.71978124295696944, -141.5628872026273086, -18.23991632971910803 ) ) ;
#12051=CARTESIAN_POINT ( 'NONE',  ( -12.32444585054070885, 42.03964062063555929, 32.41407232917325132 ) ) ;
#12055=CARTESIAN_POINT ( 'NONE',  ( -57.08002265617300708, 84.22855780814606419, 15.00000000000006573 ) ) ;
#12064=PLANE ( 'NONE',  #12044 ) ;
#12078=CARTESIAN_POINT ( 'NONE',  ( -123.4618227840623632, -151.5628872026273086, 57.00000000000000000 ) ) ;
#12092=VECTOR ( 'NONE', #4506, 1000.000000000000000 ) ;
#12094=DIRECTION ( 'NONE',  ( 0.000000000000000000, 0.000000000000000000, 1.000000000000000000 ) ) ;
#12100=DIRECTION ( 'NONE',  ( -0.000000000000000000, 0.000000000000000000, 1.000000000000000000 ) ) ;
#12109=ADVANCED_FACE ( 'NONE', ( #9964 ), #7150, .T. ) ;
#12110=ORIENTED_EDGE ( 'NONE', *, *, #11097, .T. ) ;
#12115=CARTESIAN_POINT ( 'NONE',  ( -67.59262256747319952, 110.5691553257988460, 26.35917033480641436 ) ) ;
#12125=PLANE ( 'NONE',  #2775 ) ;
#12133=ORIENTED_EDGE ( 'NONE', *, *, #9390, .F. ) ;
#12141=CARTESIAN_POINT ( 'NONE',  ( 3.411723673005281121, -3.146036035674485642, 51.39613239753626317 ) ) ;
#12150=DIRECTION ( 'NONE',  ( 1.000000000000000000, 0.000000000000000000, 0.000000000000000000 ) ) ;
#12155=EDGE_CURVE ( 'NONE', #17871, #7519, #10030, .T. ) ;
#12160=CARTESIAN_POINT ( 'NONE',  ( 103.5381772159376084, -151.5628872026272802, -57.00000000000000000 ) ) ;
#12162=CARTESIAN_POINT ( 'NONE',  ( -102.4618227840623774, 0.000000000000000000, 57.00000000000000000 ) ) ;
#12169=CARTESIAN_POINT ( 'NONE',  ( -73.17959092978806268, 59.66472505855460895, -22.77303213590205644 ) ) ;
#12185=CARTESIAN_POINT ( 'NONE',  ( -67.59262256747317110, 56.80567558672318995, -22.50837044127973030 ) ) ;
#12195=EDGE_LOOP ( 'NONE', ( #1379, #17115, #7442, #65, #721, #7677 ) ) ;
#12200=DIRECTION ( 'NONE',  ( 1.000000000000000000, 2.062304371594500494E-16, -0.000000000000000000 ) ) ;
#12204=EDGE_CURVE ( 'NONE', #8849, #6958, #14492, .T. ) ;
#12206=ORIENTED_EDGE ( 'NONE', *, *, #12576, .T. ) ;
#12209=VERTEX_POINT ( 'NONE', #7070 ) ;
#12210=FACE_BOUND ( 'NONE', #17933, .T. ) ;
#12215=DIRECTION ( 'NONE',  ( 0.000000000000000000, 0.000000000000000000, 1.000000000000000000 ) ) ;
#12220=CARTESIAN_POINT ( 'NONE',  ( 1.779151955615176695, 2.685460533711434117, 49.75286364766792957 ) ) ;
#12238=EDGE_CURVE ( 'NONE', #6083, #12209, #17771, .T. ) ;
#12241=VECTOR ( 'NONE', #7168, 1000.000000000000000 ) ;
#12243=DIRECTION ( 'NONE',  ( 0.000000000000000000, -0.000000000000000000, -1.000000000000000000 ) ) ;
#12253=DIRECTION ( 'NONE',  ( -1.000000000000000000, 0.000000000000000000, 0.000000000000000000 ) ) ;
#12256=AXIS2_PLACEMENT_3D ( 'NONE', #12548, #10755, #9741 ) ;
#12262=ORIENTED_EDGE ( 'NONE', *, *, #5589, .F. ) ;
#12280=ORIENTED_EDGE ( 'NONE', *, *, #6879, .T. ) ;
#12285=VECTOR ( 'NONE', #6783, 1000.000000000000000 ) ;
#12294=ORIENTED_EDGE ( 'NONE', *, *, #12371, .T. ) ;
#12295=AXIS2_PLACEMENT_3D ( 'NONE', #908, #284, #8900 ) ;
#12300=VECTOR ( 'NONE', #13497, 1000.000000000000000 ) ;
#12304=EDGE_LOOP ( 'NONE', ( #5682, #2572 ) ) ;
#12308=ORIENTED_EDGE ( 'NONE', *, *, #12514, .F. ) ;
#12309=CARTESIAN_POINT ( 'NONE',  ( -76.11078808681516250, 106.5972831367397333, -25.83450869657911397 ) ) ;
#12310=DIRECTION ( 'NONE',  ( -1.000000000000000000, -0.000000000000000000, -0.000000000000000000 ) ) ;
#12313=CIRCLE ( 'NONE', #1842, 29.36884788726140627 ) ;
#12325=DIRECTION ( 'NONE',  ( -1.000000000000000000, 0.000000000000000000, 0.000000000000000000 ) ) ;
#12335=CARTESIAN_POINT ( 'NONE',  ( -13.50321529758715933, 29.05444879267565739, -39.44013366681765120 ) ) ;
#12351=CARTESIAN_POINT ( 'NONE',  ( -66.40868851600845346, 56.38066346224191960, 25.00000000000000355 ) ) ;
#12353=DIRECTION ( 'NONE',  ( -0.000000000000000000, 1.000000000000000000, -1.200240087506842815E-16 ) ) ;
#12354=VECTOR ( 'NONE', #15973, 1000.000000000000000 ) ;
#12356=FACE_OUTER_BOUND ( 'NONE', #11167, .T. ) ;
#12364=AXIS2_PLACEMENT_3D ( 'NONE', #8414, #4016, #18143 ) ;
#12371=EDGE_CURVE ( 'NONE', #9953, #7618, #18241, .T. ) ;
#12372=ADVANCED_FACE ( 'NONE', ( #12356 ), #5233, .T. ) ;
#12377=CYLINDRICAL_SURFACE ( 'NONE', #5000, 3.999999999999989786 ) ;
#12379=DIRECTION ( 'NONE',  ( 1.000000000000000000, 0.000000000000000000, 0.000000000000000000 ) ) ;
#12402=CARTESIAN_POINT ( 'NONE',  ( 5.233202738124664855, -46.83756720124470263, 115.7605492041889619 ) ) ;
#12415=CARTESIAN_POINT ( 'NONE',  ( -75.72335493167709330, 106.9211863004614997, -28.00000000000000355 ) ) ;
#12424=EDGE_LOOP ( 'NONE', ( #10414, #14042, #5653, #13359, #12441, #8722, #5715, #5505, #4382, #4149, #4108, #13634, #10004, #15492, #8638, #15725 ) ) ;
#12430=DIRECTION ( 'NONE',  ( -0.000000000000000000, -0.000000000000000000, -1.000000000000000000 ) ) ;
#12440=DIRECTION ( 'NONE',  ( -1.000000000000000000, -0.000000000000000000, -0.000000000000000000 ) ) ;
#12441=ORIENTED_EDGE ( 'NONE', *, *, #4936, .F. ) ;
#12442=CARTESIAN_POINT ( 'NONE',  ( 95.45835937779679625, 56.41207303426869402, 7.000000000000010658 ) ) ;
#12446=CARTESIAN_POINT ( 'NONE',  ( -100.4870060002411805, -151.5628872026273086, -57.00000000000000000 ) ) ;
#12451=DIRECTION ( 'NONE',  ( 0.000000000000000000, 1.000000000000000000, -5.906678677474559343E-17 ) ) ;
#12453=CARTESIAN_POINT ( 'NONE',  ( 95.45835937779683888, -32.62665103886256190, -3.000000000000000000 ) ) ;
#12457=VERTEX_POINT ( 'NONE', #15141 ) ;
#12458=EDGE_CURVE ( 'NONE', #3309, #885, #10313, .T. ) ;
#12459=CARTESIAN_POINT ( 'NONE',  ( -71.67320232791250589, 58.72641804341122906, -22.41725278188095061 ) ) ;
#12469=DIRECTION ( 'NONE',  ( 1.000000000000000000, 1.119176436114069332E-16, 0.000000000000000000 ) ) ;
#12472=DIRECTION ( 'NONE',  ( -0.000000000000000000, -0.000000000000000000, -1.000000000000000000 ) ) ;
#12485=ORIENTED_EDGE ( 'NONE', *, *, #11791, .F. ) ;
#12488=ORIENTED_EDGE ( 'NONE', *, *, #12034, .F. ) ;
#12489=EDGE_CURVE ( 'NONE', #6749, #9163, #4643, .T. ) ;
#12500=EDGE_CURVE ( 'NONE', #8524, #12741, #17016, .T. ) ;
#12506=CARTESIAN_POINT ( 'NONE',  ( -86.44887054343442401, 84.22855780814606419, 15.00000000000006573 ) ) ;
#12511=ORIENTED_EDGE ( 'NONE', *, *, #8239, .T. ) ;
#12512=ORIENTED_EDGE ( 'NONE', *, *, #5725, .T. ) ;
#12514=EDGE_CURVE ( 'NONE', #8646, #4482, #15628, .T. ) ;
#12527=CARTESIAN_POINT ( 'NONE',  ( 2.393365886519067232, 0.7544924491581967985, -50.32767191113995153 ) ) ;
#12529=ORIENTED_EDGE ( 'NONE', *, *, #1640, .F. ) ;
#12539=CARTESIAN_POINT ( 'NONE',  ( -74.91216001386696632, 60.89270028045363858, 23.71611839326908466 ) ) ;
#12540=CARTESIAN_POINT ( 'NONE',  ( -66.30191238934644105, 56.61994693357914343, 24.99999999999999289 ) ) ;
#12542=DIRECTION ( 'NONE',  ( -1.119176436114069332E-16, 1.000000000000000000, 0.000000000000000000 ) ) ;
#12548=CARTESIAN_POINT ( 'NONE',  ( -57.08002265617300708, 84.22855780814606419, 37.50000000000000000 ) ) ;
#12554=ORIENTED_EDGE ( 'NONE', *, *, #8841, .T. ) ;
#12558=LINE ( 'NONE', #7049, #12958 ) ;
#12562=CARTESIAN_POINT ( 'NONE',  ( 5.233202738124664855, -111.0842361345572158, -57.00000000000000000 ) ) ;
#12565=EDGE_LOOP ( 'NONE', ( #18255, #1049, #16969, #5853 ) ) ;
#12566=CARTESIAN_POINT ( 'NONE',  ( -31.03642545851250745, 84.22855780814606419, -35.00000000000000711 ) ) ;
#12569=ORIENTED_EDGE ( 'NONE', *, *, #14986, .F. ) ;
#12576=EDGE_CURVE ( 'NONE', #7519, #7091, #10182, .T. ) ;
#12589=VECTOR ( 'NONE', #1474, 1000.000000000000000 ) ;
#12595=VECTOR ( 'NONE', #90, 1000.000000000000000 ) ;
#12596=EDGE_CURVE ( 'NONE', #4188, #12009, #8529, .T. ) ;
#12611=CIRCLE ( 'NONE', #14665, 3.999999999999989786 ) ;
#12613=DIRECTION ( 'NONE',  ( -0.000000000000000000, -0.000000000000000000, -1.000000000000000000 ) ) ;
#12614=CARTESIAN_POINT ( 'NONE',  ( -123.4618227840623632, -151.5628872026273086, -36.00000000000000000 ) ) ;
#12618=LINE ( 'NONE', #7088, #14028 ) ;
#12621=VERTEX_POINT ( 'NONE', #4934 ) ;
#12625=CARTESIAN_POINT ( 'NONE',  ( -75.02147910882627002, 107.4816543220079410, 23.80484796140106596 ) ) ;
#12627=CARTESIAN_POINT ( 'NONE',  ( -123.4618227840623632, -151.5628872026273086, 57.00000000000000000 ) ) ;
#12635=LINE ( 'NONE', #9722, #17038 ) ;
#12637=ORIENTED_EDGE ( 'NONE', *, *, #14546, .F. ) ;
#12642=AXIS2_PLACEMENT_3D ( 'NONE', #4713, #10081, #17265 ) ;
#12645=DIRECTION ( 'NONE',  ( -0.000000000000000000, -0.000000000000000000, -1.000000000000000000 ) ) ;
#12648=CARTESIAN_POINT ( 'NONE',  ( -66.51364668169603078, 112.0410723289543995, -28.00000000000000355 ) ) ;
#12660=VERTEX_POINT ( 'NONE', #16333 ) ;
#12664=DIRECTION ( 'NONE',  ( 0.000000000000000000, 0.000000000000000000, 1.000000000000000000 ) ) ;
#12665=DIRECTION ( 'NONE',  ( -4.124608743189000987E-16, 1.000000000000000000, 0.000000000000000000 ) ) ;
#12678=LINE ( 'NONE', #3017, #10751 ) ;
#12681=ORIENTED_EDGE ( 'NONE', *, *, #1599, .T. ) ;
#12683=VECTOR ( 'NONE', #12353, 1000.000000000000000 ) ;
#12685=ORIENTED_EDGE ( 'NONE', *, *, #11233, .T. ) ;
#12705=CARTESIAN_POINT ( 'NONE',  ( -66.34462916520553222, 56.35920651190240704, -27.54481102119680003 ) ) ;
#12711=ORIENTED_EDGE ( 'NONE', *, *, #2651, .F. ) ;
#12721=CIRCLE ( 'NONE', #9412, 172.7605492041889477 ) ;
#12733=CARTESIAN_POINT ( 'NONE',  ( 124.5381772159375942, -111.0842361345572158, 7.000000000000010658 ) ) ;
#12736=ORIENTED_EDGE ( 'NONE', *, *, #10168, .T. ) ;
#12737=EDGE_CURVE ( 'NONE', #2102, #885, #9061, .T. ) ;
#12741=VERTEX_POINT ( 'NONE', #16522 ) ;
#12759=ORIENTED_EDGE ( 'NONE', *, *, #10190, .F. ) ;
#12763=DIRECTION ( 'NONE',  ( -1.119176436114069332E-16, 1.000000000000000000, 0.000000000000000000 ) ) ;
#12764=DIRECTION ( 'NONE',  ( -0.000000000000000000, -1.000000000000000000, -0.000000000000000000 ) ) ;
#12770=FACE_OUTER_BOUND ( 'NONE', #4734, .T. ) ;
#12776=LINE ( 'NONE', #17056, #10281 ) ;
#12777=DIRECTION ( 'NONE',  ( -0.5150380749100562650, 1.049727191138617217E-16, -0.8571673007021111124 ) ) ;
#12781=CARTESIAN_POINT ( 'NONE',  ( -32.62048503522395038, 55.23029653342705814, -23.63796962397022838 ) ) ;
#12786=DIRECTION ( 'NONE',  ( -0.000000000000000000, -0.000000000000000000, -1.000000000000000000 ) ) ;
#12792=CARTESIAN_POINT ( 'NONE',  ( -100.4870060002411805, -151.5628872026273086, -57.00000000000000000 ) ) ;
#12795=LINE ( 'NONE', #12614, #11760 ) ;
#12799=CARTESIAN_POINT ( 'NONE',  ( 49.38736944425944841, -141.5628872026273086, 57.00000000000000000 ) ) ;
#12801=ORIENTED_EDGE ( 'NONE', *, *, #16664, .F. ) ;
#12805=ORIENTED_EDGE ( 'NONE', *, *, #3418, .F. ) ;
#12824=ORIENTED_EDGE ( 'NONE', *, *, #8997, .T. ) ;
#12825=EDGE_CURVE ( 'NONE', #4352, #3936, #11020, .T. ) ;
#12831=MANIFOLD_SOLID_BREP ( 'Move Face6', #15367 ) ;
#12835=ORIENTED_EDGE ( 'NONE', *, *, #2665, .T. ) ;
#12840=EDGE_CURVE ( 'NONE', #9223, #16505, #10882, .T. ) ;
#12846=CARTESIAN_POINT ( 'NONE',  ( -31.03642545851250745, 84.22855780814606419, 37.50000000000000000 ) ) ;
#12850=ORIENTED_EDGE ( 'NONE', *, *, #15594, .F. ) ;
#12857=ORIENTED_EDGE ( 'NONE', *, *, #1507, .T. ) ;
#12859=VECTOR ( 'NONE', #8268, 1000.000000000000000 ) ;
#12860=EDGE_LOOP ( 'NONE', ( #17500, #4977, #3913, #12637, #7242, #8861 ) ) ;
#12862=DIRECTION ( 'NONE',  ( 1.000000000000000000, -0.000000000000000000, -0.000000000000000000 ) ) ;
#12865=ORIENTED_EDGE ( 'NONE', *, *, #12371, .F. ) ;
#12872=ORIENTED_EDGE ( 'NONE', *, *, #8272, .F. ) ;
#12875=ORIENTED_EDGE ( 'NONE', *, *, #6841, .F. ) ;
#12876=AXIS2_PLACEMENT_3D ( 'NONE', #10299, #3185, #10382 ) ;
#12902=DIRECTION ( 'NONE',  ( -0.000000000000000000, 0.000000000000000000, 1.000000000000000000 ) ) ;
#12915=ORIENTED_EDGE ( 'NONE', *, *, #13113, .T. ) ;
#12916=CARTESIAN_POINT ( 'NONE',  ( -92.59262256747319952, 50.58224449241410525, 35.00000000000000000 ) ) ;
#12917=VECTOR ( 'NONE', #268, 1000.000000000000000 ) ;
#12925=ORIENTED_EDGE ( 'NONE', *, *, #2665, .F. ) ;
#12934=AXIS2_PLACEMENT_3D ( 'NONE', #17772, #5234, #2326 ) ;
#12945=ORIENTED_EDGE ( 'NONE', *, *, #3549, .T. ) ;
#12954=CARTESIAN_POINT ( 'NONE',  ( 49.38736944425943420, -141.5628872026273086, -57.00000000000000000 ) ) ;
#12958=VECTOR ( 'NONE', #12665, 1000.000000000000000 ) ;
#12961=LINE ( 'NONE', #13048, #2232 ) ;
#12971=FACE_OUTER_BOUND ( 'NONE', #6275, .T. ) ;
#12973=EDGE_LOOP ( 'NONE', ( #4714, #7158, #4512, #1447, #3507, #1216, #236 ) ) ;
#12981=DIRECTION ( 'NONE',  ( -0.000000000000000000, -0.000000000000000000, -1.000000000000000000 ) ) ;
#12985=LINE ( 'NONE', #10150, #12241 ) ;
#12986=DIRECTION ( 'NONE',  ( 0.000000000000000000, 0.000000000000000000, 1.000000000000000000 ) ) ;
#12993=DIRECTION ( 'NONE',  ( 4.124608743189000987E-16, -1.000000000000000000, 0.000000000000000000 ) ) ;
#12997=AXIS2_PLACEMENT_3D ( 'NONE', #2676, #14002, #15685 ) ;
#13006=CIRCLE ( 'NONE', #15058, 172.7605492041889477 ) ;
#13007=CARTESIAN_POINT ( 'NONE',  ( -64.09025127992788384, 50.58224449241410525, 28.00000000000000355 ) ) ;
#13013=CARTESIAN_POINT ( 'NONE',  ( -92.59262256747321373, 117.8748711238780373, 35.00000000000000000 ) ) ;
#13014=CIRCLE ( 'NONE', #4917, 29.36884788726140627 ) ;
#13027=ORIENTED_EDGE ( 'NONE', *, *, #16947, .F. ) ;
#13033=LINE ( 'NONE', #4492, #6613 ) ;
#13036=ORIENTED_EDGE ( 'NONE', *, *, #9273, .F. ) ;
#13046=EDGE_CURVE ( 'NONE', #6830, #7572, #7026, .T. ) ;
#13047=ORIENTED_EDGE ( 'NONE', *, *, #5010, .T. ) ;
#13048=CARTESIAN_POINT ( 'NONE',  ( -123.4618227840623632, -111.0842361345572158, -57.00000000000000000 ) ) ;
#13052=ORIENTED_EDGE ( 'NONE', *, *, #1227, .T. ) ;
#13054=ORIENTED_EDGE ( 'NONE', *, *, #4109, .F. ) ;
#13056=DIRECTION ( 'NONE',  ( -1.000000000000000000, 0.000000000000000000, 0.000000000000000000 ) ) ;
#13057=DIRECTION ( 'NONE',  ( 0.000000000000000000, 0.000000000000000000, 1.000000000000000000 ) ) ;
#13060=ORIENTED_EDGE ( 'NONE', *, *, #1705, .F. ) ;
#13065=EDGE_CURVE ( 'NONE', #6083, #9555, #1377, .T. ) ;
#13073=EDGE_CURVE ( 'NONE', #6976, #16629, #16914, .T. ) ;
#13094=CARTESIAN_POINT ( 'NONE',  ( -69.66239992860627694, 84.22855780814606419, 25.00000000000000355 ) ) ;
#13104=VECTOR ( 'NONE', #13688, 1000.000000000000000 ) ;
#13110=LINE ( 'NONE', #550, #13154 ) ;
#13113=EDGE_CURVE ( 'NONE', #12209, #12621, #13910, .T. ) ;
#13118=ORIENTED_EDGE ( 'NONE', *, *, #5496, .F. ) ;
#13122=ORIENTED_EDGE ( 'NONE', *, *, #8841, .F. ) ;
#13129=CARTESIAN_POINT ( 'NONE',  ( -50.06979403241810900, 50.58224449241409104, 26.91246033477412425 ) ) ;
#13131=DIRECTION ( 'NONE',  ( 0.000000000000000000, -0.000000000000000000, -1.000000000000000000 ) ) ;
#13141=CARTESIAN_POINT ( 'NONE',  ( -57.08002265617300708, 84.22855780814606419, 37.50000000000000000 ) ) ;
#13144=EDGE_CURVE ( 'NONE', #3936, #4543, #4355, .T. ) ;
#13146=CARTESIAN_POINT ( 'NONE',  ( 276.3098885457529832, -32.62665103886256190, -7.000000000000010658 ) ) ;
#13154=VECTOR ( 'NONE', #5974, 1000.000000000000000 ) ;
#13162=PLANE ( 'NONE',  #11352 ) ;
#13172=EDGE_CURVE ( 'NONE', #16713, #13980, #7937, .T. ) ;
#13175=CARTESIAN_POINT ( 'NONE',  ( -66.17173038963701970, 112.1547175742259697, -26.82650548119792688 ) ) ;
#13176=CARTESIAN_POINT ( 'NONE',  ( -67.59262256747315689, 111.6514400295689313, 37.50000000000000000 ) ) ;
#13188=CARTESIAN_POINT ( 'NONE',  ( -67.59262256747317110, 61.64996188551982215, 25.00000000000000355 ) ) ;
#13202=CARTESIAN_POINT ( 'NONE',  ( -64.09025127992791226, 117.8748711238780373, 28.00000000000000355 ) ) ;
#13215=ORIENTED_EDGE ( 'NONE', *, *, #6514, .F. ) ;
#13218=CARTESIAN_POINT ( 'NONE',  ( -45.07652969643970664, 51.92630754768256907, -25.99113068039098451 ) ) ;
#13232=AXIS2_PLACEMENT_3D ( 'NONE', #12115, #16390, #2187 ) ;
#13238=CARTESIAN_POINT ( 'NONE',  ( 15.23320273812466041, -19.34983604512934363, 54.79921157549236455 ) ) ;
#13240=ORIENTED_EDGE ( 'NONE', *, *, #3189, .T. ) ;
#13242=DIRECTION ( 'NONE',  ( 1.000000000000000000, 0.000000000000000000, 0.000000000000000000 ) ) ;
#13247=AXIS2_PLACEMENT_3D ( 'NONE', #6345, #10753, #6247 ) ;
#13248=CIRCLE ( 'NONE', #9656, 34.36884788726141693 ) ;
#13253=FACE_BOUND ( 'NONE', #1080, .T. ) ;
#13264=DIRECTION ( 'NONE',  ( -0.000000000000000000, -0.000000000000000000, 1.000000000000000000 ) ) ;
#13266=ORIENTED_EDGE ( 'NONE', *, *, #1852, .F. ) ;
#13268=EDGE_CURVE ( 'NONE', #14752, #15269, #6090, .T. ) ;
#13279=CARTESIAN_POINT ( 'NONE',  ( 15.23320273812466574, -111.0842361345572158, 57.00000000000000000 ) ) ;
#13288=ORIENTED_EDGE ( 'NONE', *, *, #13113, .F. ) ;
#13298=PLANE ( 'NONE',  #8731 ) ;
#13301=DIRECTION ( 'NONE',  ( 1.000000000000000000, 0.000000000000000000, 0.000000000000000000 ) ) ;
#13304=AXIS2_PLACEMENT_3D ( 'NONE', #16177, #13383, #17674 ) ;
#13305=PLANE ( 'NONE',  #13304 ) ;
#13311=ORIENTED_EDGE ( 'NONE', *, *, #2651, .T. ) ;
#13316=MECHANICAL_DESIGN_GEOMETRIC_PRESENTATION_REPRESENTATION('',(#11822),#14505);
#13317=VECTOR ( 'NONE', #10367, 1000.000000000000000 ) ;
#13319=CARTESIAN_POINT ( 'NONE',  ( 15.23320273812467462, -111.0842361345572158, 3.000000000000000000 ) ) ;
#13328=ORIENTED_EDGE ( 'NONE', *, *, #8250, .T. ) ;
#13355=CARTESIAN_POINT ( 'NONE',  ( -92.59262256747319952, 57.88796029049329661, -22.35917033480642502 ) ) ;
#13359=ORIENTED_EDGE ( 'NONE', *, *, #414, .F. ) ;
#13363=LINE ( 'NONE', #17760, #1232 ) ;
#13369=CARTESIAN_POINT ( 'NONE',  ( -57.08002265617300708, 84.22855780814606419, 28.00000000000000355 ) ) ;
#13372=DIRECTION ( 'NONE',  ( 0.000000000000000000, 0.000000000000000000, -1.000000000000000000 ) ) ;
#13380=CARTESIAN_POINT ( 'NONE',  ( -76.04777162888156283, 61.80621309083046100, -27.19272967165976596 ) ) ;
#13383=DIRECTION ( 'NONE',  ( -1.000000000000000000, 0.000000000000000000, 0.000000000000000000 ) ) ;
#13386=AXIS2_PLACEMENT_3D ( 'NONE', #11715, #14522, #3110 ) ;
#13404=VERTEX_POINT ( 'NONE', #12442 ) ;
#13409=ORIENTED_EDGE ( 'NONE', *, *, #457, .F. ) ;
#13411=VERTEX_POINT ( 'NONE', #9807 ) ;
#13418=CARTESIAN_POINT ( 'NONE',  ( -68.12361985383350316, 84.22855780814606419, -47.49999999999999289 ) ) ;
#13419=EDGE_LOOP ( 'NONE', ( #18010, #1091, #16021, #14394, #9436, #16757 ) ) ;
#13426=CIRCLE ( 'NONE', #8657, 26.04359719766049608 ) ;
#13436=VECTOR ( 'NONE', #12764, 1000.000000000000000 ) ;
#13442=VERTEX_POINT ( 'NONE', #14118 ) ;
#13445=CARTESIAN_POINT ( 'NONE',  ( -112.5926225674731995, 50.58224449241410525, -35.00000000000000000 ) ) ;
#13455=VECTOR ( 'NONE', #14036, 1000.000000000000000 ) ;
#13462=ORIENTED_EDGE ( 'NONE', *, *, #4855, .F. ) ;
#13463=CYLINDRICAL_SURFACE ( 'NONE', #6719, 3.999999999999996447 ) ;
#13471=FACE_OUTER_BOUND ( 'NONE', #10260, .T. ) ;
#13472=VERTEX_POINT ( 'NONE', #10083 ) ;
#13475=CARTESIAN_POINT ( 'NONE',  ( -75.94240647281702650, 61.71752694572068521, -25.18301127684852858 ) ) ;
#13490=VERTEX_POINT ( 'NONE', #7180 ) ;
#13496=FACE_OUTER_BOUND ( 'NONE', #5698, .T. ) ;
#13497=DIRECTION ( 'NONE',  ( 0.000000000000000000, -1.000000000000000000, 0.000000000000000000 ) ) ;
#13501=AXIS2_PLACEMENT_3D ( 'NONE', #139, #11556, #13057 ) ;
#13517=DIRECTION ( 'NONE',  ( -0.000000000000000000, -0.000000000000000000, -1.000000000000000000 ) ) ;
#13525=CARTESIAN_POINT ( 'NONE',  ( -66.00585202009864361, 110.3988717985813395, 25.00000000000000355 ) ) ;
#13535=ORIENTED_EDGE ( 'NONE', *, *, #8363, .F. ) ;
#13548=EDGE_LOOP ( 'NONE', ( #9459, #14550 ) ) ;
#13558=CARTESIAN_POINT ( 'NONE',  ( -70.85175816390371040, -141.5628872026273086, 18.23991632971911514 ) ) ;
#13562=CARTESIAN_POINT ( 'NONE',  ( -66.00585202009801833, 57.88796029049324687, 25.00000000000000355 ) ) ;
#13564=AXIS2_PLACEMENT_3D ( 'NONE', #17011, #8319, #7108 ) ;
#13573=AXIS2_PLACEMENT_3D ( 'NONE', #5072, #17990, #4983 ) ;
#13580=ORIENTED_EDGE ( 'NONE', *, *, #1599, .F. ) ;
#13581=PRODUCT_DEFINITION_CONTEXT ( 'detailed design', #15160, 'design' ) ;
#13583=LINE ( 'NONE', #10865, #6401 ) ;
#13597=AXIS2_PLACEMENT_3D ( 'NONE', #15341, #16445, #12253 ) ;
#13615=CARTESIAN_POINT ( 'NONE',  ( -70.06856178257680767, 110.5691553257988460, 22.35917033480641791 ) ) ;
#13619=DIRECTION ( 'NONE',  ( -0.000000000000000000, -0.000000000000000000, -1.000000000000000000 ) ) ;
#13623=FACE_BOUND ( 'NONE', #16579, .T. ) ;
#13624=EDGE_CURVE ( 'NONE', #5660, #8650, #6403, .T. ) ;
#13631=EDGE_LOOP ( 'NONE', ( #11524, #3081, #2366, #7698 ) ) ;
#13632=LINE ( 'NONE', #9421, #7282 ) ;
#13634=ORIENTED_EDGE ( 'NONE', *, *, #3423, .F. ) ;
#13639=ORIENTED_EDGE ( 'NONE', *, *, #11525, .F. ) ;
#13648=EDGE_CURVE ( 'NONE', #3936, #565, #14214, .T. ) ;
#13649=ORIENTED_EDGE ( 'NONE', *, *, #6750, .T. ) ;
#13656=CARTESIAN_POINT ( 'NONE',  ( -67.59262256747315689, 56.80567558672318285, -15.00000000000000711 ) ) ;
#13657=CARTESIAN_POINT ( 'NONE',  ( -72.31238267408940601, 59.11671001647612655, 22.54839013747459120 ) ) ;
#13664=ADVANCED_FACE ( 'NONE', ( #13623, #12210, #14730 ), #10527, .F. ) ;
#13672=FACE_BOUND ( 'NONE', #6096, .T. ) ;
#13681=CARTESIAN_POINT ( 'NONE',  ( -57.08002265617300708, 84.22855780814606419, -15.00000000000000711 ) ) ;
#13682=DIRECTION ( 'NONE',  ( 1.000000000000000000, 0.000000000000000000, 0.000000000000000000 ) ) ;
#13683=VERTEX_POINT ( 'NONE', #12030 ) ;
#13685=VERTEX_POINT ( 'NONE', #6202 ) ;
#13688=DIRECTION ( 'NONE',  ( -1.000000000000000000, -0.000000000000000000, -0.000000000000000000 ) ) ;
#13690=ORIENTED_EDGE ( 'NONE', *, *, #3512, .T. ) ;
#13702=CARTESIAN_POINT ( 'NONE',  ( -73.18550356302633020, 108.7913366739104646, -22.76494920255247578 ) ) ;
#13706=DIRECTION ( 'NONE',  ( -2.062304371594500494E-16, 1.000000000000000000, 0.000000000000000000 ) ) ;
#13708=DIRECTION ( 'NONE',  ( -1.000000000000000000, 0.000000000000000000, 0.000000000000000000 ) ) ;
#13716=CARTESIAN_POINT ( 'NONE',  ( -7.398807083024507847, 21.35709021097153482, 42.97347408463063090 ) ) ;
#13718=DIRECTION ( 'NONE',  ( 0.000000000000000000, -1.000000000000000000, 0.000000000000000000 ) ) ;
#13726=EDGE_CURVE ( 'NONE', #8524, #1462, #15401, .T. ) ;
#13727=ADVANCED_FACE ( 'NONE', ( #15293 ), #5370, .F. ) ;
#13736=EDGE_LOOP ( 'NONE', ( #6642, #8292, #8119, #18510, #2948, #6136, #399, #7109, #8652, #8286, #11045 ) ) ;
#13738=VECTOR ( 'NONE', #4439, 1000.000000000000000 ) ;
#13743=CARTESIAN_POINT ( 'NONE',  ( -73.88125023881575260, 60.13841621731533849, 23.04531203040799525 ) ) ;
#13745=CARTESIAN_POINT ( 'NONE',  ( -66.26741375599719674, 58.64497179233082846, -28.00000000000000000 ) ) ;
#13759=PLANE ( 'NONE',  #16377 ) ;
#13761=ORIENTED_EDGE ( 'NONE', *, *, #14261, .T. ) ;
#13763=CIRCLE ( 'NONE', #15844, 26.04359719766049608 ) ;
#13764=ORIENTED_EDGE ( 'NONE', *, *, #14625, .F. ) ;
#13767=DIRECTION ( 'NONE',  ( -1.000000000000000000, -0.000000000000000000, -0.000000000000000000 ) ) ;
#13772=CARTESIAN_POINT ( 'NONE',  ( -75.86129610575210336, 106.8071537307722991, 25.00000000000000355 ) ) ;
#13775=DIRECTION ( 'NONE',  ( 0.000000000000000000, 1.000000000000000000, -5.906678677474559343E-17 ) ) ;
#13781=ORIENTED_EDGE ( 'NONE', *, *, #1407, .T. ) ;
#13795=ORIENTED_EDGE ( 'NONE', *, *, #13268, .T. ) ;
#13800=CARTESIAN_POINT ( 'NONE',  ( -75.86088625105277572, 106.8078580376686944, -24.98227212054766611 ) ) ;
#13802=ORIENTED_EDGE ( 'NONE', *, *, #4597, .T. ) ;
#13816=CARTESIAN_POINT ( 'NONE',  ( -92.59262256747321373, 117.8748711238780373, 35.00000000000000000 ) ) ;
#13817=CARTESIAN_POINT ( 'NONE',  ( 113.3630170098442989, -111.0842361345572158, 3.000000000000000000 ) ) ;
#13823=CARTESIAN_POINT ( 'NONE',  ( -0.2208807544345702534, 8.409232685097855153, -47.97696181894473710 ) ) ;
#13829=VERTEX_POINT ( 'NONE', #8290 ) ;
#13841=DIRECTION ( 'NONE',  ( 0.000000000000000000, 0.000000000000000000, 1.000000000000000000 ) ) ;
#13846=DIRECTION ( 'NONE',  ( 1.000000000000000000, 0.000000000000000000, 0.000000000000000000 ) ) ;
#13867=LINE ( 'NONE', #1059, #8530 ) ;
#13873=APPLICATION_CONTEXT ( 'automotive_design' ) ;
#13874=EDGE_LOOP ( 'NONE', ( #9749, #15669, #12554, #6253, #14745 ) ) ;
#13880=LINE ( 'NONE', #15373, #12859 ) ;
#13889=AXIS2_PLACEMENT_3D ( 'NONE', #8757, #788, #7703 ) ;
#13891=DIRECTION ( 'NONE',  ( -0.000000000000000000, -0.000000000000000000, -1.000000000000000000 ) ) ;
#13892=DIRECTION ( 'NONE',  ( 0.000000000000000000, 0.000000000000000000, -1.000000000000000000 ) ) ;
#13898=CARTESIAN_POINT ( 'NONE',  ( 13.61986053733008184, -2.650911626341202254, -51.30709107799135182 ) ) ;
#13901=DIRECTION ( 'NONE',  ( 1.000000000000000000, 0.000000000000000000, 0.000000000000000000 ) ) ;
#13905=CARTESIAN_POINT ( 'NONE',  ( -75.94242511790328365, 106.7395705226562654, -25.18349236146325865 ) ) ;
#13910=LINE ( 'NONE', #8384, #7304 ) ;
#13911=VECTOR ( 'NONE', #7380, 1000.000000000000000 ) ;
#13928=CARTESIAN_POINT ( 'NONE',  ( 5.233202738124671960, -15.17993412113254337, -54.12718235529279553 ) ) ;
#13933=DIRECTION ( 'NONE',  ( -1.000000000000000000, -0.000000000000000000, -0.000000000000000000 ) ) ;
#13934=DIRECTION ( 'NONE',  ( -0.9475106458593564041, -0.3197242186372270534, 0.000000000000000000 ) ) ;
#13940=LINE ( 'NONE', #8128, #10263 ) ;
#13954=ADVANCED_FACE ( 'NONE', ( #6251 ), #13305, .F. ) ;
#13959=CARTESIAN_POINT ( 'NONE',  ( -57.08002265617300708, 84.22855780814606419, 35.00000000000000000 ) ) ;
#13963=FACE_OUTER_BOUND ( 'NONE', #5906, .T. ) ;
#13975=B_SPLINE_CURVE_WITH_KNOTS ( 'NONE', 3,
 ( #10911, #13525, #3789, #2199, #16601, #3700, #608, #7633, #16315, #6486, #17725, #9491 ),
 .UNSPECIFIED., .F., .F.,
 ( 4, 2, 2, 2, 2, 4 ),
 ( 0.009411782824043968959, 0.009923328437046213812, 0.01043487405004845693, 0.01145796527605294490, 0.01248105650205743287, 0.01350414772806192085 ),
 .UNSPECIFIED. ) ;
#13980=VERTEX_POINT ( 'NONE', #3275 ) ;
#13988=ORIENTED_EDGE ( 'NONE', *, *, #14225, .F. ) ;
#13990=CARTESIAN_POINT ( 'NONE',  ( 12.67459307379139233, 1.374362345496204174, -50.18803144527930016 ) ) ;
#13995=CARTESIAN_POINT ( 'NONE',  ( -68.43470539589056045, 111.3286264100576801, 22.41764221539786917 ) ) ;
#13998=CARTESIAN_POINT ( 'NONE',  ( -57.08002265617300708, 84.22855780814606419, 25.00000000000000355 ) ) ;
#14002=DIRECTION ( 'NONE',  ( 1.000000000000000000, 2.062304371594500494E-16, -0.000000000000000000 ) ) ;
#14017=CARTESIAN_POINT ( 'NONE',  ( -16.92216393104348171, 32.58739983099662396, -37.66730993204898681 ) ) ;
#14018=CARTESIAN_POINT ( 'NONE',  ( 13.61981611287037808, -2.650921210901910463, 51.30707055644251824 ) ) ;
#14021=CARTESIAN_POINT ( 'NONE',  ( -92.59262256747321373, 117.8748711238780373, -15.00000000000000711 ) ) ;
#14028=VECTOR ( 'NONE', #16696, 1000.000000000000000 ) ;
#14030=EDGE_CURVE ( 'NONE', #7906, #10991, #15246, .T. ) ;
#14036=DIRECTION ( 'NONE',  ( -0.000000000000000000, -0.000000000000000000, 1.000000000000000000 ) ) ;
#14042=ORIENTED_EDGE ( 'NONE', *, *, #6841, .T. ) ;
#14043=DIRECTION ( 'NONE',  ( -1.000000000000000000, -0.000000000000000000, -0.000000000000000000 ) ) ;
#14049=DIRECTION ( 'NONE',  ( -0.000000000000000000, 1.000000000000000000, -0.000000000000000000 ) ) ;
#14056=VECTOR ( 'NONE', #17014, 1000.000000000000000 ) ;
#14062=CARTESIAN_POINT ( 'NONE',  ( -65.18918009136295666, 110.5691553257988318, 26.35917033480641436 ) ) ;
#14063=ORIENTED_EDGE ( 'NONE', *, *, #678, .T. ) ;
#14066=CIRCLE ( 'NONE', #14363, 3.999999999999989786 ) ;
#14073=LINE ( 'NONE', #8461, #10562 ) ;
#14075=EDGE_CURVE ( 'NONE', #12741, #16981, #18059, .T. ) ;
#14082=DIRECTION ( 'NONE',  ( -6.608470384673552010E-16, 0.000000000000000000, -1.000000000000000000 ) ) ;
#14089=DIRECTION ( 'NONE',  ( -1.000000000000000000, -0.000000000000000000, 1.156482317317869999E-16 ) ) ;
#14090=EDGE_LOOP ( 'NONE', ( #17787, #7435, #15392, #11729, #5406 ) ) ;
#14113=CARTESIAN_POINT ( 'NONE',  ( -15.52181756281650493, 31.21008990100222391, -38.37361753973598155 ) ) ;
#14114=CARTESIAN_POINT ( 'NONE',  ( 12.67495189244583287, 1.372358515719736882, 50.18853589267851589 ) ) ;
#14118=CARTESIAN_POINT ( 'NONE',  ( -64.09025127992791226, 109.3109350805793270, 35.00000000000000000 ) ) ;
#14120=CARTESIAN_POINT ( 'NONE',  ( -92.59262256747319952, 57.88796029049329661, -26.35917033480641436 ) ) ;
#14127=AXIS2_PLACEMENT_3D ( 'NONE', #7116, #9486, #16059 ) ;
#14142=CARTESIAN_POINT ( 'NONE',  ( -57.08002265617300708, 84.22855780814606419, 15.00000000000006573 ) ) ;
#14144=ORIENTED_EDGE ( 'NONE', *, *, #4636, .T. ) ;
#14170=CARTESIAN_POINT ( 'NONE',  ( -67.59262256747319952, 110.5691553257988460, 22.35917033480642502 ) ) ;
#14176=CARTESIAN_POINT ( 'NONE',  ( -9.438806153496912543, 39.35910582506906508, -33.99713577918199547 ) ) ;
#14177=DIRECTION ( 'NONE',  ( 0.000000000000000000, 0.000000000000000000, 1.000000000000000000 ) ) ;
#14180=DIRECTION ( 'NONE',  ( 1.000000000000000000, 0.000000000000000000, 0.000000000000000000 ) ) ;
#14188=CARTESIAN_POINT ( 'NONE',  ( -123.4618227840623632, -151.5628872026273086, 57.00000000000000000 ) ) ;
#14194=ADVANCED_FACE ( 'NONE', ( #1904 ), #15531, .T. ) ;
#14200=EDGE_LOOP ( 'NONE', ( #2632, #16524, #10912, #4329, #7798, #543, #1259, #17358 ) ) ;
#14202=CARTESIAN_POINT ( 'NONE',  ( -127.5926225674731711, 61.53592931583062864, -28.00000000000000355 ) ) ;
#14203=CARTESIAN_POINT ( 'NONE',  ( -83.12361985383350316, 84.22855780814606419, 37.50000000000000000 ) ) ;
#14207=ORIENTED_EDGE ( 'NONE', *, *, #4242, .F. ) ;
#14208=EDGE_CURVE ( 'NONE', #6726, #2809, #16842, .T. ) ;
#14211=CARTESIAN_POINT ( 'NONE',  ( 3.839657907260265013, -5.121192436768893685, -51.90027309438220016 ) ) ;
#14212=PLANE ( 'NONE',  #6025 ) ;
#14214=CIRCLE ( 'NONE', #4330, 3.999999999999989786 ) ;
#14225=EDGE_CURVE ( 'NONE', #2768, #17254, #10919, .T. ) ;
#14232=ORIENTED_EDGE ( 'NONE', *, *, #5172, .F. ) ;
#14251=CARTESIAN_POINT ( 'NONE',  ( 79.02261728059691848, -151.5628872026273086, -57.00000000000000000 ) ) ;
#14253=PLANE ( 'NONE',  #1546 ) ;
#14261=EDGE_CURVE ( 'NONE', #5721, #6695, #3345, .T. ) ;
#14263=LINE ( 'NONE', #6860, #430 ) ;
#14283=CARTESIAN_POINT ( 'NONE',  ( -127.5926225674731995, 110.5691553257988460, -26.35917033480641436 ) ) ;
#14284=CARTESIAN_POINT ( 'NONE',  ( -64.09025127992791226, 117.8748711238780373, -35.00000000000000000 ) ) ;
#14294=ORIENTED_EDGE ( 'NONE', *, *, #11215, .F. ) ;
#14299=CARTESIAN_POINT ( 'NONE',  ( -31.03642545851250745, 84.22855780814606419, 37.50000000000000000 ) ) ;
#14302=VERTEX_POINT ( 'NONE', #8973 ) ;
#14314=CARTESIAN_POINT ( 'NONE',  ( 113.3630170098443273, -111.0842361345571874, 7.000000000000010658 ) ) ;
#14315=DIRECTION ( 'NONE',  ( 0.000000000000000000, 0.000000000000000000, 1.000000000000000000 ) ) ;
#14323=ORIENTED_EDGE ( 'NONE', *, *, #16366, .F. ) ;
#14326=ADVANCED_FACE ( 'NONE', ( #6618, #16429 ), #741, .T. ) ;
#14328=DIRECTION ( 'NONE',  ( 1.000000000000000000, 4.675871521838984962E-16, -0.000000000000000000 ) ) ;
#14329=CARTESIAN_POINT ( 'NONE',  ( -123.4618227840623632, -151.5628872026273086, 57.00000000000000000 ) ) ;
#14341=PLANE ( 'NONE',  #15491 ) ;
#14348=ORIENTED_EDGE ( 'NONE', *, *, #10190, .T. ) ;
#14351=DIRECTION ( 'NONE',  ( -0.000000000000000000, -0.000000000000000000, -1.000000000000000000 ) ) ;
#14363=AXIS2_PLACEMENT_3D ( 'NONE', #16153, #637, #10556 ) ;
#14364=DIRECTION ( 'NONE',  ( 0.000000000000000000, 0.000000000000000000, 1.000000000000000000 ) ) ;
#14371=CARTESIAN_POINT ( 'NONE',  ( -86.44887054343442401, 84.22855780814606419, 37.50000000000000000 ) ) ;
#14378=VECTOR ( 'NONE', #301, 1000.000000000000000 ) ;
#14382=VECTOR ( 'NONE', #16878, 1000.000000000000000 ) ;
#14394=ORIENTED_EDGE ( 'NONE', *, *, #6495, .F. ) ;
#14397=CIRCLE ( 'NONE', #6305, 26.04359719766049608 ) ;
#14408=DIRECTION ( 'NONE',  ( -0.000000000000000000, -0.000000000000000000, -1.000000000000000000 ) ) ;
#14415=AXIS2_PLACEMENT_3D ( 'NONE', #7651, #10994, #6687 ) ;
#14420=DIRECTION ( 'NONE',  ( -0.000000000000000000, -0.000000000000000000, 1.000000000000000000 ) ) ;
#14422=CYLINDRICAL_SURFACE ( 'NONE', #3010, 20.99999999999999645 ) ;
#14430=CARTESIAN_POINT ( 'NONE',  ( 5.233202738124664855, -111.0842361345572158, 57.00000000000000000 ) ) ;
#14435=VERTEX_POINT ( 'NONE', #4943 ) ;
#14438=EDGE_CURVE ( 'NONE', #13404, #3088, #16340, .T. ) ;
#14439=VECTOR ( 'NONE', #12472, 1000.000000000000000 ) ;
#14445=CARTESIAN_POINT ( 'NONE',  ( 5.233202738124664855, -46.83756720124470263, -115.7605492041889619 ) ) ;
#14451=LINE ( 'NONE', #4257, #9591 ) ;
#14454=EDGE_CURVE ( 'NONE', #12621, #3501, #12635, .T. ) ;
#14457=VECTOR ( 'NONE', #10423, 1000.000000000000000 ) ;
#14460=CYLINDRICAL_SURFACE ( 'NONE', #10273, 81.86696747278379860 ) ;
#14461=DIRECTION ( 'NONE',  ( 1.000000000000000000, 0.000000000000000000, -0.000000000000000000 ) ) ;
#14467=AXIS2_PLACEMENT_3D ( 'NONE', #10487, #4767, #6262 ) ;
#14474=ORIENTED_EDGE ( 'NONE', *, *, #7769, .F. ) ;
#14484=EDGE_CURVE ( 'NONE', #11504, #1708, #8977, .T. ) ;
#14491=CARTESIAN_POINT ( 'NONE',  ( 124.5381772159375942, -111.0842361345572158, -6.999999999999985789 ) ) ;
#14492=CIRCLE ( 'NONE', #6729, 26.04359719766049608 ) ;
#14497=VERTEX_POINT ( 'NONE', #8595 ) ;
#14505=( GEOMETRIC_REPRESENTATION_CONTEXT ( 3 ) GLOBAL_UNCERTAINTY_ASSIGNED_CONTEXT ( ( #14876 ) ) GLOBAL_UNIT_ASSIGNED_CONTEXT ( ( #3998, #5393, #7933 ) ) REPRESENTATION_CONTEXT ( 'NONE', 'WORKASPACE' ) );
#14508=EDGE_CURVE ( 'NONE', #1462, #2272, #11227, .T. ) ;
#14513=LINE ( 'NONE', #11440, #4812 ) ;
#14514=EDGE_LOOP ( 'NONE', ( #11844, #17490, #5244, #9111, #14294, #9458, #9976 ) ) ;
#14517=CARTESIAN_POINT ( 'NONE',  ( -66.40868851600848188, 112.0764521540501875, 25.00000000000000355 ) ) ;
#14522=DIRECTION ( 'NONE',  ( -0.000000000000000000, -0.000000000000000000, -1.000000000000000000 ) ) ;
#14526=EDGE_CURVE ( 'NONE', #17119, #7091, #9809, .T. ) ;
#14533=DIRECTION ( 'NONE',  ( -0.000000000000000000, -0.000000000000000000, -1.000000000000000000 ) ) ;
#14546=EDGE_CURVE ( 'NONE', #7091, #15955, #3909, .T. ) ;
#14548=EDGE_CURVE ( 'NONE', #6499, #15744, #3861, .T. ) ;
#14550=ORIENTED_EDGE ( 'NONE', *, *, #14863, .F. ) ;
#14551=LINE ( 'NONE', #14202, #13738 ) ;
#14555=EDGE_LOOP ( 'NONE', ( #15918, #2506, #9139, #486, #9209, #11007, #13988, #13266, #2267, #11334 ) ) ;
#14562=ORIENTED_EDGE ( 'NONE', *, *, #14075, .T. ) ;
#14568=( NAMED_UNIT ( * ) PLANE_ANGLE_UNIT ( ) SI_UNIT ( $, .RADIAN. ) );
#14583=ORIENTED_EDGE ( 'NONE', *, *, #14030, .T. ) ;
#14591=CARTESIAN_POINT ( 'NONE',  ( 276.3098885457529832, -32.62665103886256190, 7.000000000000010658 ) ) ;
#14594=ORIENTED_EDGE ( 'NONE', *, *, #16707, .T. ) ;
#14596=CARTESIAN_POINT ( 'NONE',  ( -67.59262256747315689, 129.5689604715732912, 15.00000000000005862 ) ) ;
#14602=ORIENTED_EDGE ( 'NONE', *, *, #1705, .T. ) ;
#14612=DIRECTION ( 'NONE',  ( 0.000000000000000000, -1.000000000000000000, 0.000000000000000000 ) ) ;
#14619=CARTESIAN_POINT ( 'NONE',  ( 95.45835937779683888, -32.62665103886256190, 7.000000000000010658 ) ) ;
#14620=ORIENTED_EDGE ( 'NONE', *, *, #12825, .T. ) ;
#14624=ADVANCED_FACE ( 'NONE', ( #13253, #17194 ), #9044, .F. ) ;
#14625=EDGE_CURVE ( 'NONE', #5721, #6138, #11584, .T. ) ;
#14630=DIRECTION ( 'NONE',  ( -0.000000000000000000, -0.000000000000000000, -1.000000000000000000 ) ) ;
#14645=CIRCLE ( 'NONE', #11079, 29.36884788726140627 ) ;
#14649=VERTEX_POINT ( 'NONE', #16128 ) ;
#14650=ADVANCED_FACE ( 'NONE', ( #7638 ), #13162, .F. ) ;
#14651=AXIS2_PLACEMENT_3D ( 'NONE', #186, #4390, #10098 ) ;
#14665=AXIS2_PLACEMENT_3D ( 'NONE', #791, #12200, #17892 ) ;
#14668=CARTESIAN_POINT ( 'NONE',  ( -66.32174931794583017, 59.21973273998174392, 25.00000000000000711 ) ) ;
#14681=CARTESIAN_POINT ( 'NONE',  ( -57.08002265617300708, 84.22855780814606419, 37.50000000000000000 ) ) ;
#14682=ORIENTED_EDGE ( 'NONE', *, *, #10891, .T. ) ;
#14684=LINE ( 'NONE', #14596, #10252 ) ;
#14691=EDGE_LOOP ( 'NONE', ( #46, #18471, #13690, #15848, #11900 ) ) ;
#14695=CARTESIAN_POINT ( 'NONE',  ( -36.44155368744860368, 56.74635804676025685, -22.50216374311546019 ) ) ;
#14701=ORIENTED_EDGE ( 'NONE', *, *, #13648, .T. ) ;
#14705=DIRECTION ( 'NONE',  ( -0.000000000000000000, 1.000000000000000000, -0.000000000000000000 ) ) ;
#14707=CARTESIAN_POINT ( 'NONE',  ( -36.44155368744860368, 56.74635804676025685, -22.50216374311546019 ) ) ;
#14722=ORIENTED_EDGE ( 'NONE', *, *, #17152, .T. ) ;
#14730=FACE_OUTER_BOUND ( 'NONE', #15547, .T. ) ;
#14732=ORIENTED_EDGE ( 'NONE', *, *, #14755, .F. ) ;
#14745=ORIENTED_EDGE ( 'NONE', *, *, #727, .T. ) ;
#14748=DIRECTION ( 'NONE',  ( -0.000000000000000000, 1.000000000000000000, -0.000000000000000000 ) ) ;
#14749=DIRECTION ( 'NONE',  ( 1.000000000000000000, 0.000000000000000000, 0.000000000000000000 ) ) ;
#14752=VERTEX_POINT ( 'NONE', #5090 ) ;
#14754=EDGE_CURVE ( 'NONE', #7519, #748, #14824, .T. ) ;
#14755=EDGE_CURVE ( 'NONE', #2330, #299, #1530, .T. ) ;
#14758=AXIS2_PLACEMENT_3D ( 'NONE', #11894, #9371, #15069 ) ;
#14759=DIRECTION ( 'NONE',  ( 0.000000000000000000, -1.000000000000000000, 1.181335735494911869E-16 ) ) ;
#14760=ORIENTED_EDGE ( 'NONE', *, *, #14754, .F. ) ;
#14766=AXIS2_PLACEMENT_3D ( 'NONE', #1927, #7637, #13706 ) ;
#14769=EDGE_CURVE ( 'NONE', #15127, #2177, #10808, .T. ) ;
#14772=CARTESIAN_POINT ( 'NONE',  ( -57.08002265617300708, 84.22855780814606419, -28.00000000000000355 ) ) ;
#14780=CARTESIAN_POINT ( 'NONE',  ( -75.72335493167710752, 61.53592931583062864, -28.00000000000000355 ) ) ;
#14788=ORIENTED_EDGE ( 'NONE', *, *, #11176, .T. ) ;
#14821=DIRECTION ( 'NONE',  ( -2.062304371594500494E-16, 1.000000000000000000, 0.000000000000000000 ) ) ;
#14824=LINE ( 'NONE', #4996, #5659 ) ;
#14840=CYLINDRICAL_SURFACE ( 'NONE', #12029, 180.8515291679561585 ) ;
#14846=ORIENTED_EDGE ( 'NONE', *, *, #2182, .T. ) ;
#14853=EDGE_CURVE ( 'NONE', #15127, #5660, #2683, .T. ) ;
#14856=CARTESIAN_POINT ( 'NONE',  ( 124.5381772159375942, -46.83756720124470263, 57.00000000000000000 ) ) ;
#14863=EDGE_CURVE ( 'NONE', #15269, #14752, #13426, .T. ) ;
#14865=CARTESIAN_POINT ( 'NONE',  ( -76.14500017491396022, 61.88899956654809387, -26.29040544024000425 ) ) ;
#14872=VERTEX_POINT ( 'NONE', #15301 ) ;
#14876=UNCERTAINTY_MEASURE_WITH_UNIT (LENGTH_MEASURE( 1.000000000000000082E-05 ), #3998, 'distance_accuracy_value', 'NONE');
#14877=ADVANCED_FACE ( 'NONE', ( #9598 ), #11013, .T. ) ;
#14878=CYLINDRICAL_SURFACE ( 'NONE', #9075, 172.7605492041889477 ) ;
#14911=VERTEX_POINT ( 'NONE', #18312 ) ;
#14928=FACE_OUTER_BOUND ( 'NONE', #1753, .T. ) ;
#14935=ORIENTED_EDGE ( 'NONE', *, *, #12737, .T. ) ;
#14936=B_SPLINE_CURVE_WITH_KNOTS ( 'NONE', 3,
 ( #9349, #16539, #9530, #15046, #929, #16720, #13745, #3919, #15233, #2240, #10949, #18045, #2521, #18238 ),
 .UNSPECIFIED., .F., .F.,
 ( 4, 2, 2, 2, 2, 2, 4 ),
 ( 0.01646133141517134441, 0.01782527105796415101, 0.01918921070075695762, 0.01987118052215335745, 0.02021216543285155390, 0.02055315034354975381, 0.02191708998634258124 ),
 .UNSPECIFIED. ) ;
#14938=AXIS2_PLACEMENT_3D ( 'NONE', #12446, #18138, #13934 ) ;
#14945=ADVANCED_FACE ( 'NONE', ( #2494 ), #5201, .F. ) ;
#14947=CIRCLE ( 'NONE', #15559, 12.58237727243326987 ) ;
#14951=CARTESIAN_POINT ( 'NONE',  ( -76.06859087019410026, 61.82386385984740684, -25.61244817148770991 ) ) ;
#14965=CARTESIAN_POINT ( 'NONE',  ( -65.18918009136292824, 57.88796029049328240, 26.35917033480641436 ) ) ;
#14975=CARTESIAN_POINT ( 'NONE',  ( -66.40868851600848188, 112.0764521540501875, 25.00000000000000355 ) ) ;
#14977=DIRECTION ( 'NONE',  ( 0.000000000000000000, 0.000000000000000000, 1.000000000000000000 ) ) ;
#14979=CIRCLE ( 'NONE', #17660, 3.999999999999989786 ) ;
#14986=EDGE_CURVE ( 'NONE', #17238, #7705, #12985, .T. ) ;
#14991=VECTOR ( 'NONE', #12993, 1000.000000000000000 ) ;
#14992=VECTOR ( 'NONE', #6826, 1000.000000000000000 ) ;
#14993=CARTESIAN_POINT ( 'NONE',  ( -92.59262256747319952, 57.88796029049329661, 30.35917033480640370 ) ) ;
#14996=CARTESIAN_POINT ( 'NONE',  ( -67.59262256747319952, 110.5691553257988460, 26.35917033480641436 ) ) ;
#15001=LINE ( 'NONE', #16216, #1816 ) ;
#15023=CARTESIAN_POINT ( 'NONE',  ( 276.3098885457529832, -32.62665103886256190, 7.000000000000010658 ) ) ;
#15025=LINE ( 'NONE', #9329, #2111 ) ;
#15028=CARTESIAN_POINT ( 'NONE',  ( -28.94822502443852841, 53.44157543122878451, 24.93952570249303946 ) ) ;
#15046=CARTESIAN_POINT ( 'NONE',  ( -66.75451753366466789, 59.92410785088754466, -28.00000000000000000 ) ) ;
#15049=AXIS2_PLACEMENT_3D ( 'NONE', #3806, #3894, #18022 ) ;
#15050=DIRECTION ( 'NONE',  ( 0.000000000000000000, -1.000000000000000000, -0.000000000000000000 ) ) ;
#15051=CIRCLE ( 'NONE', #1618, 95.91469608272775815 ) ;
#15056=CYLINDRICAL_SURFACE ( 'NONE', #12256, 11.04359719766049430 ) ;
#15058=AXIS2_PLACEMENT_3D ( 'NONE', #2466, #12862, #16869 ) ;
#15064=VECTOR ( 'NONE', #9347, 1000.000000000000000 ) ;
#15069=DIRECTION ( 'NONE',  ( 1.000000000000000000, 0.000000000000000000, 0.000000000000000000 ) ) ;
#15088=EDGE_CURVE ( 'NONE', #14649, #15284, #14551, .T. ) ;
#15089=ORIENTED_EDGE ( 'NONE', *, *, #8250, .F. ) ;
#15092=AXIS2_PLACEMENT_3D ( 'NONE', #530, #6222, #6132 ) ;
#15102=DIRECTION ( 'NONE',  ( 0.000000000000000000, 0.000000000000000000, 1.000000000000000000 ) ) ;
#15105=ORIENTED_EDGE ( 'NONE', *, *, #1852, .T. ) ;
#15113=ADVANCED_FACE ( 'NONE', ( #9989 ), #11939, .F. ) ;
#15118=ORIENTED_EDGE ( 'NONE', *, *, #14438, .T. ) ;
#15120=CARTESIAN_POINT ( 'NONE',  ( -5.756396797216070560, 18.89541522413301067, 44.01604086321188447 ) ) ;
#15123=DIRECTION ( 'NONE',  ( -0.000000000000000000, 1.000000000000000000, -0.000000000000000000 ) ) ;
#15124=LINE ( 'NONE', #1010, #15407 ) ;
#15126=CARTESIAN_POINT ( 'NONE',  ( -70.85175816390371040, -141.5628872026273086, -57.00000000000000000 ) ) ;
#15127=VERTEX_POINT ( 'NONE', #16564 ) ;
#15141=CARTESIAN_POINT ( 'NONE',  ( -46.03642545851251100, 84.22855780814606419, -28.00000000000000355 ) ) ;
#15142=DIRECTION ( 'NONE',  ( -0.000000000000000000, 0.000000000000000000, 1.000000000000000000 ) ) ;
#15160=APPLICATION_CONTEXT ( 'automotive_design' ) ;
#15169=ORIENTED_EDGE ( 'NONE', *, *, #10075, .T. ) ;
#15193=ADVANCED_FACE ( 'NONE', ( #2164 ), #9193, .F. ) ;
#15194=EDGE_CURVE ( 'NONE', #3213, #4188, #6364, .T. ) ;
#15196=ORIENTED_EDGE ( 'NONE', *, *, #5390, .T. ) ;
#15217=ORIENTED_EDGE ( 'NONE', *, *, #3925, .T. ) ;
#15225=ORIENTED_EDGE ( 'NONE', *, *, #2932, .F. ) ;
#15232=CARTESIAN_POINT ( 'NONE',  ( -75.01613753673549922, 60.97256703306408809, 23.80938688424596350 ) ) ;
#15233=CARTESIAN_POINT ( 'NONE',  ( -66.19006831724836104, 58.19665835547753119, -27.99999999999999645 ) ) ;
#15237=DIRECTION ( 'NONE',  ( 1.000000000000000000, 0.000000000000000000, 0.000000000000000000 ) ) ;
#15238=ORIENTED_EDGE ( 'NONE', *, *, #3089, .T. ) ;
#15241=CARTESIAN_POINT ( 'NONE',  ( -70.88454472225026848, 58.29032118345796931, -22.35917033480642502 ) ) ;
#15242=AXIS2_PLACEMENT_3D ( 'NONE', #4116, #2525, #8233 ) ;
#15243=VECTOR ( 'NONE', #14408, 1000.000000000000000 ) ;
#15246=LINE ( 'NONE', #6542, #1067 ) ;
#15250=AXIS2_PLACEMENT_3D ( 'NONE', #11146, #18154, #10854 ) ;
#15255=LINE ( 'NONE', #2442, #18066 ) ;
#15266=AXIS2_PLACEMENT_3D ( 'NONE', #496, #14533, #10601 ) ;
#15269=VERTEX_POINT ( 'NONE', #1240 ) ;
#15283=LINE ( 'NONE', #16673, #8197 ) ;
#15284=VERTEX_POINT ( 'NONE', #2835 ) ;
#15285=FACE_OUTER_BOUND ( 'NONE', #13631, .T. ) ;
#15291=VERTEX_POINT ( 'NONE', #15740 ) ;
#15293=FACE_OUTER_BOUND ( 'NONE', #1347, .T. ) ;
#15301=CARTESIAN_POINT ( 'NONE',  ( 5.233202738124664855, -111.0842361345572158, -57.00000000000000000 ) ) ;
#15322=EDGE_CURVE ( 'NONE', #7705, #14872, #8442, .T. ) ;
#15338=CARTESIAN_POINT ( 'NONE',  ( -31.03642545851250745, 84.22855780814606419, 28.00000000000000355 ) ) ;
#15340=LINE ( 'NONE', #838, #6409 ) ;
#15341=CARTESIAN_POINT ( 'NONE',  ( -57.08002265617300708, 84.22855780814606419, 37.50000000000000000 ) ) ;
#15342=DIRECTION ( 'NONE',  ( 1.558623840612994987E-16, 1.000000000000000000, 0.000000000000000000 ) ) ;
#15346=AXIS2_PLACEMENT_3D ( 'NONE', #1382, #5294, #16792 ) ;
#15367=CLOSED_SHELL ( 'NONE', ( #7673, #15552, #951, #3210, #5740, #570, #4630, #6493, #7543, #10204, #12372, #8260, #1628, #13664, #712, #3440, #10639, #17455, #17285, #14877, #2779, #2273, #18121, #16580, #8473, #81, #487, #14194, #16680, #9961, #802, #13954, #10636, #11641, #1841, #13727, #15710, #10006, #9519, #6709, #7102, #2085, #11583, #4460, #4464, #15193, #5607, #1710, #2065, #10387, #2063, #14624, #561, #1700, #2292, #18407, #17604, #14650, #144, #2308, #6246, #4677, #15908, #15461, #15554, #12109, #7841, #5940, #9391, #9911, #14326, #3772, #7213, #14945, #3102, #9499, #11990, #5147, #15113, #16811, #9385, #2769, #27, #9728, #8929 ) ) ;
#15373=CARTESIAN_POINT ( 'NONE',  ( -127.5926225674731711, 57.88796029049329661, 22.35917033480642502 ) ) ;
#15387=ORIENTED_EDGE ( 'NONE', *, *, #3189, .F. ) ;
#15390=CARTESIAN_POINT ( 'NONE',  ( -28.96456321416951596, 53.44918566155911321, -24.93391072407674613 ) ) ;
#15392=ORIENTED_EDGE ( 'NONE', *, *, #11920, .F. ) ;
#15395=PLANE ( 'NONE',  #6645 ) ;
#15401=LINE ( 'NONE', #15587, #16872 ) ;
#15407=VECTOR ( 'NONE', #2501, 1000.000000000000000 ) ;
#15422=CARTESIAN_POINT ( 'NONE',  ( 9.727308505134775629, 10.18372637758682764, 47.32161794854564363 ) ) ;
#15426=DIRECTION ( 'NONE',  ( 0.000000000000000000, 1.000000000000000000, 0.000000000000000000 ) ) ;
#15431=PLANE ( 'NONE',  #5175 ) ;
#15433=FACE_OUTER_BOUND ( 'NONE', #13736, .T. ) ;
#15437=DIRECTION ( 'NONE',  ( -0.000000000000000000, -0.000000000000000000, -1.000000000000000000 ) ) ;
#15439=CARTESIAN_POINT ( 'NONE',  ( -100.4870060002411805, -151.5628872026273086, -57.00000000000000000 ) ) ;
#15455=CYLINDRICAL_SURFACE ( 'NONE', #9388, 3.999999999999989786 ) ;
#15456=LINE ( 'NONE', #2445, #14439 ) ;
#15461=ADVANCED_FACE ( 'NONE', ( #17302 ), #4670, .T. ) ;
#15466=EDGE_CURVE ( 'NONE', #748, #7603, #13110, .T. ) ;
#15483=FACE_OUTER_BOUND ( 'NONE', #12860, .T. ) ;
#15485=CARTESIAN_POINT ( 'NONE',  ( -73.90245058923942167, 108.3059858121137182, -23.04901498212743505 ) ) ;
#15489=CARTESIAN_POINT ( 'NONE',  ( -66.51364668169601657, 56.41604328733773599, -28.00000000000000355 ) ) ;
#15491=AXIS2_PLACEMENT_3D ( 'NONE', #15829, #8826, #4594 ) ;
#15492=ORIENTED_EDGE ( 'NONE', *, *, #13073, .F. ) ;
#15506=VERTEX_POINT ( 'NONE', #10469 ) ;
#15509=DIRECTION ( 'NONE',  ( -0.000000000000000000, -0.000000000000000000, -1.000000000000000000 ) ) ;
#15514=DIRECTION ( 'NONE',  ( 1.000000000000000000, 0.000000000000000000, -0.000000000000000000 ) ) ;
#15521=CARTESIAN_POINT ( 'NONE',  ( -67.15738250865011594, 107.7249262104797225, -28.00000000000000355 ) ) ;
#15531=CYLINDRICAL_SURFACE ( 'NONE', #6570, 172.7605492041889192 ) ;
#15537=CARTESIAN_POINT ( 'NONE',  ( -70.06856178257687873, 57.88796029049330372, -22.35917033480642502 ) ) ;
#15539=VECTOR ( 'NONE', #5137, 1000.000000000000000 ) ;
#15547=EDGE_LOOP ( 'NONE', ( #10111, #18227, #10860, #16724 ) ) ;
#15550=CYLINDRICAL_SURFACE ( 'NONE', #15831, 95.91469608272775815 ) ;
#15552=ADVANCED_FACE ( 'NONE', ( #204 ), #11704, .F. ) ;
#15554=ADVANCED_FACE ( 'NONE', ( #4749 ), #14422, .T. ) ;
#15557=ORIENTED_EDGE ( 'NONE', *, *, #8572, .T. ) ;
#15559=AXIS2_PLACEMENT_3D ( 'NONE', #16056, #7290, #1489 ) ;
#15560=EDGE_CURVE ( 'NONE', #7091, #7155, #9878, .T. ) ;
#15573=DIRECTION ( 'NONE',  ( 0.000000000000000000, 0.000000000000000000, 1.000000000000000000 ) ) ;
#15582=ORIENTED_EDGE ( 'NONE', *, *, #3545, .F. ) ;
#15587=CARTESIAN_POINT ( 'NONE',  ( -92.59262256747321373, 117.8748711238780373, 35.00000000000000000 ) ) ;
#15594=EDGE_CURVE ( 'NONE', #15506, #10929, #8382, .T. ) ;
#15601=CARTESIAN_POINT ( 'NONE',  ( -50.06979403241810900, 50.58224449241409104, 26.91246033477412425 ) ) ;
#15606=CARTESIAN_POINT ( 'NONE',  ( -12.84402433037575442, 28.32093258747478615, -39.79682189825760474 ) ) ;
#15622=CARTESIAN_POINT ( 'NONE',  ( -66.51167281958223043, 112.0421917453874556, -24.67744962832335176 ) ) ;
#15626=LINE ( 'NONE', #7112, #5965 ) ;
#15627=CARTESIAN_POINT ( 'NONE',  ( -67.59262256747317110, 57.88796029049329661, 22.35917033480642857 ) ) ;
#15628=LINE ( 'NONE', #14314, #9132 ) ;
#15633=ORIENTED_EDGE ( 'NONE', *, *, #12458, .F. ) ;
#15639=ORIENTED_EDGE ( 'NONE', *, *, #12034, .T. ) ;
#15644=AXIS2_PLACEMENT_3D ( 'NONE', #8255, #10869, #11056 ) ;
#15645=CARTESIAN_POINT ( 'NONE',  ( -68.43244712042248068, 57.12762349320347965, -22.41788552795556910 ) ) ;
#15657=DIRECTION ( 'NONE',  ( -1.000000000000000000, 0.000000000000000000, 0.000000000000000000 ) ) ;
#15660=EDGE_LOOP ( 'NONE', ( #177, #9658, #16867, #1608, #2099, #13036 ) ) ;
#15668=EDGE_LOOP ( 'NONE', ( #3911, #9503, #3555, #8094 ) ) ;
#15669=ORIENTED_EDGE ( 'NONE', *, *, #14454, .T. ) ;
#15676=CIRCLE ( 'NONE', #4886, 34.36884788726141693 ) ;
#15685=DIRECTION ( 'NONE',  ( 0.000000000000000000, 1.000000000000000000, 0.000000000000000000 ) ) ;
#15700=CARTESIAN_POINT ( 'NONE',  ( -24.42865639074866735, 38.95740195071884671, 34.21208529195362047 ) ) ;
#15703=EDGE_CURVE ( 'NONE', #14497, #18083, #5231, .T. ) ;
#15710=ADVANCED_FACE ( 'NONE', ( #11324 ), #3920, .F. ) ;
#15713=EDGE_CURVE ( 'NONE', #1208, #14302, #18149, .T. ) ;
#15725=ORIENTED_EDGE ( 'NONE', *, *, #10694, .F. ) ;
#15737=LINE ( 'NONE', #2919, #2848 ) ;
#15740=CARTESIAN_POINT ( 'NONE',  ( 15.23320273812467462, -111.0842361345572158, -57.00000000000000000 ) ) ;
#15744=VERTEX_POINT ( 'NONE', #15338 ) ;
#15760=CARTESIAN_POINT ( 'NONE',  ( -70.85175816390371040, -141.5628872026273086, -57.00000000000000000 ) ) ;
#15761=ORIENTED_EDGE ( 'NONE', *, *, #8372, .T. ) ;
#15769=EDGE_CURVE ( 'NONE', #9327, #14302, #2906, .T. ) ;
#15775=DIRECTION ( 'NONE',  ( -0.000000000000000000, -0.000000000000000000, -1.000000000000000000 ) ) ;
#15785=DIRECTION ( 'NONE',  ( 1.000000000000000000, 0.000000000000000000, -0.000000000000000000 ) ) ;
#15789=EDGE_CURVE ( 'NONE', #7618, #2809, #9566, .T. ) ;
#15797=DIRECTION ( 'NONE',  ( 0.000000000000000000, 1.000000000000000000, 0.000000000000000000 ) ) ;
#15800=LINE ( 'NONE', #15627, #11543 ) ;
#15801=DIRECTION ( 'NONE',  ( 1.000000000000000000, 0.000000000000000000, 0.000000000000000000 ) ) ;
#15806=EDGE_CURVE ( 'NONE', #17762, #3055, #16987, .T. ) ;
#15813=VERTEX_POINT ( 'NONE', #5602 ) ;
#15817=EDGE_CURVE ( 'NONE', #11585, #17119, #15626, .T. ) ;
#15826=AXIS2_PLACEMENT_3D ( 'NONE', #5864, #7539, #15785 ) ;
#15829=CARTESIAN_POINT ( 'NONE',  ( 15.23320273812466574, -111.0842361345572158, 57.00000000000000000 ) ) ;
#15831=AXIS2_PLACEMENT_3D ( 'NONE', #5633, #11355, #15657 ) ;
#15841=CARTESIAN_POINT ( 'NONE',  ( -36.44155368744862500, 56.74635804676027107, 2.999999999999999112 ) ) ;
#15844=AXIS2_PLACEMENT_3D ( 'NONE', #6326, #2035, #6137 ) ;
#15846=EDGE_LOOP ( 'NONE', ( #3279, #7397, #16186, #10217, #6073, #9909, #2570 ) ) ;
#15848=ORIENTED_EDGE ( 'NONE', *, *, #255, .T. ) ;
#15849=VECTOR ( 'NONE', #5773, 1000.000000000000000 ) ;
#15851=ORIENTED_EDGE ( 'NONE', *, *, #6750, .F. ) ;
#15854=CYLINDRICAL_SURFACE ( 'NONE', #6689, 3.999999999999996447 ) ;
#15861=DIRECTION ( 'NONE',  ( 1.000000000000000000, 0.000000000000000000, 0.000000000000000000 ) ) ;
#15867=CIRCLE ( 'NONE', #10780, 11.04359719766049430 ) ;
#15872=ORIENTED_EDGE ( 'NONE', *, *, #3512, .F. ) ;
#15891=ORIENTED_EDGE ( 'NONE', *, *, #9268, .T. ) ;
#15900=EDGE_CURVE ( 'NONE', #1479, #14497, #14947, .T. ) ;
#15908=ADVANCED_FACE ( 'NONE', ( #9058 ), #7197, .F. ) ;
#15910=DIRECTION ( 'NONE',  ( -0.000000000000000000, -0.000000000000000000, -1.000000000000000000 ) ) ;
#15912=EDGE_CURVE ( 'NONE', #8070, #9559, #5954, .T. ) ;
#15918=ORIENTED_EDGE ( 'NONE', *, *, #9852, .F. ) ;
#15925=ORIENTED_EDGE ( 'NONE', *, *, #4109, .T. ) ;
#15937=DIRECTION ( 'NONE',  ( -1.000000000000000000, -0.000000000000000000, -0.000000000000000000 ) ) ;
#15946=DIRECTION ( 'NONE',  ( -1.000000000000000000, -0.000000000000000000, -0.000000000000000000 ) ) ;
#15947=DIRECTION ( 'NONE',  ( 1.000000000000000000, 0.000000000000000000, 0.000000000000000000 ) ) ;
#15955=VERTEX_POINT ( 'NONE', #14491 ) ;
#15969=ORIENTED_EDGE ( 'NONE', *, *, #17580, .T. ) ;
#15971=VECTOR ( 'NONE', #3119, 1000.000000000000000 ) ;
#15972=DIRECTION ( 'NONE',  ( -1.000000000000000000, -0.000000000000000000, -0.000000000000000000 ) ) ;
#15973=DIRECTION ( 'NONE',  ( -0.5150380749100570421, 0.000000000000000000, 0.8571673007021106683 ) ) ;
#15975=ORIENTED_EDGE ( 'NONE', *, *, #15560, .F. ) ;
#15997=CARTESIAN_POINT ( 'NONE',  ( -50.41499038512539954, 117.9449492212793444, 7.000000000000010658 ) ) ;
#16001=DIRECTION ( 'NONE',  ( -1.000000000000000000, -0.000000000000000000, -0.000000000000000000 ) ) ;
#16003=DIRECTION ( 'NONE',  ( -5.204170427930409450E-16, 0.000000000000000000, 1.000000000000000000 ) ) ;
#16008=EDGE_CURVE ( 'NONE', #535, #9559, #15025, .T. ) ;
#16020=EDGE_CURVE ( 'NONE', #293, #4298, #10187, .T. ) ;
#16021=ORIENTED_EDGE ( 'NONE', *, *, #12737, .F. ) ;
#16036=FACE_OUTER_BOUND ( 'NONE', #18383, .T. ) ;
#16038=CARTESIAN_POINT ( 'NONE',  ( 124.5381772159375942, -111.0842361345572158, -35.99999999999997158 ) ) ;
#16056=CARTESIAN_POINT ( 'NONE',  ( -57.08002265617300708, 84.22855780814606419, 25.00000000000000355 ) ) ;
#16059=DIRECTION ( 'NONE',  ( 1.000000000000000000, 0.000000000000000000, 0.000000000000000000 ) ) ;
#16062=VERTEX_POINT ( 'NONE', #2303 ) ;
#16081=VECTOR ( 'NONE', #11811, 1000.000000000000000 ) ;
#16084=CARTESIAN_POINT ( 'NONE',  ( -68.43628269749412141, 57.12909386699050884, 22.41747227276118792 ) ) ;
#16088=CIRCLE ( 'NONE', #8944, 29.36884788726140627 ) ;
#16093=AXIS2_PLACEMENT_3D ( 'NONE', #804, #16504, #13708 ) ;
#16096=CARTESIAN_POINT ( 'NONE',  ( -66.00585202009864361, 110.8305070361169840, 25.00000000000000355 ) ) ;
#16114=ORIENTED_EDGE ( 'NONE', *, *, #13172, .T. ) ;
#16121=ORIENTED_EDGE ( 'NONE', *, *, #4410, .T. ) ;
#16122=CARTESIAN_POINT ( 'NONE',  ( -50.41499038512538533, 117.9449492212793444, 2.999999999999999112 ) ) ;
#16128=CARTESIAN_POINT ( 'NONE',  ( -75.72335493167710752, 61.53592931583062864, -28.00000000000000355 ) ) ;
#16153=CARTESIAN_POINT ( 'NONE',  ( -67.59262256747319952, 110.5691553257988460, -26.35917033480641436 ) ) ;
#16154=VERTEX_POINT ( 'NONE', #3996 ) ;
#16164=CARTESIAN_POINT ( 'NONE',  ( -70.64221740337633548, 110.2804215074198737, 22.36668740498762276 ) ) ;
#16165=DIRECTION ( 'NONE',  ( 0.000000000000000000, 1.000000000000000000, 0.000000000000000000 ) ) ;
#16177=CARTESIAN_POINT ( 'NONE',  ( 15.23320273812466574, -111.0842361345572158, 57.00000000000000000 ) ) ;
#16179=FACE_OUTER_BOUND ( 'NONE', #2673, .T. ) ;
#16181=ORIENTED_EDGE ( 'NONE', *, *, #12489, .T. ) ;
#16185=CARTESIAN_POINT ( 'NONE',  ( -92.59262256747319952, 50.58224449241410525, -15.00000000000000178 ) ) ;
#16186=ORIENTED_EDGE ( 'NONE', *, *, #11249, .T. ) ;
#16201=ORIENTED_EDGE ( 'NONE', *, *, #5725, .F. ) ;
#16206=AXIS2_PLACEMENT_3D ( 'NONE', #8263, #18267, #5441 ) ;
#16208=CARTESIAN_POINT ( 'NONE',  ( -92.59262256747321373, 110.5691553257988460, -30.35917033480641081 ) ) ;
#16216=CARTESIAN_POINT ( 'NONE',  ( -70.85175816390371040, -141.5628872026273086, 57.00000000000000000 ) ) ;
#16217=AXIS2_PLACEMENT_3D ( 'NONE', #5781, #6037, #8961 ) ;
#16218=VECTOR ( 'NONE', #1814, 1000.000000000000000 ) ;
#16236=EDGE_CURVE ( 'NONE', #12009, #16154, #1824, .T. ) ;
#16244=CYLINDRICAL_SURFACE ( 'NONE', #16894, 29.36884788726140627 ) ;
#16247=FACE_OUTER_BOUND ( 'NONE', #2463, .T. ) ;
#16253=CIRCLE ( 'NONE', #9110, 81.86696747278378439 ) ;
#16271=CARTESIAN_POINT ( 'NONE',  ( -70.06856178257680767, 110.5691553257988460, 22.35917033480641791 ) ) ;
#16278=ORIENTED_EDGE ( 'NONE', *, *, #12155, .T. ) ;
#16285=DIRECTION ( 'NONE',  ( 0.000000000000000000, 0.000000000000000000, 1.000000000000000000 ) ) ;
#16315=CARTESIAN_POINT ( 'NONE',  ( -66.92854697799583619, 108.0100032524460261, 25.00000000000000355 ) ) ;
#16333=CARTESIAN_POINT ( 'NONE',  ( -123.4618227840623632, -111.0842361345572158, 36.00000000000001421 ) ) ;
#16336=EDGE_CURVE ( 'NONE', #9679, #4169, #7174, .T. ) ;
#16340=LINE ( 'NONE', #3528, #4197 ) ;
#16352=CARTESIAN_POINT ( 'NONE',  ( -70.35643127740523539, 110.4272069818263446, 22.35917033480641436 ) ) ;
#16357=DIRECTION ( 'NONE',  ( 0.000000000000000000, 0.000000000000000000, -1.000000000000000000 ) ) ;
#16359=CARTESIAN_POINT ( 'NONE',  ( -75.29929411668209127, 61.19352203925132017, -24.09877121037940739 ) ) ;
#16366=EDGE_CURVE ( 'NONE', #8650, #8537, #15001, .T. ) ;
#16369=DIRECTION ( 'NONE',  ( 1.000000000000000000, 0.000000000000000000, -0.000000000000000000 ) ) ;
#16371=CARTESIAN_POINT ( 'NONE',  ( -40.55373863553682412, 54.08738549153932951, -24.45531647972368461 ) ) ;
#16377=AXIS2_PLACEMENT_3D ( 'NONE', #6543, #946, #6646 ) ;
#16382=ORIENTED_EDGE ( 'NONE', *, *, #7655, .F. ) ;
#16386=ORIENTED_EDGE ( 'NONE', *, *, #7763, .F. ) ;
#16390=DIRECTION ( 'NONE',  ( -1.000000000000000000, -0.000000000000000000, -0.000000000000000000 ) ) ;
#16394=ORIENTED_EDGE ( 'NONE', *, *, #10168, .F. ) ;
#16396=B_SPLINE_CURVE_WITH_KNOTS ( 'NONE', 3,
 ( #9584, #5565, #6876, #2284, #9783, #883, #13702, #15485, #987, #16600, #7988, #3788, #2372, #8083, #1272, #13800, #13905, #6586, #12309, #18003, #3972, #5190, #10910, #8187, #1096, #12415 ),
 .UNSPECIFIED., .F., .F.,
 ( 4, 2, 2, 2, 2, 2, 2, 2, 2, 2, 2, 2, 4 ),
 ( 0.002699315152504066541, 0.004048330729320218091, 0.005397346306136370508, 0.006746361882952522059, 0.008095377459768675343, 0.008769885248176737674, 0.009444393036584803475, 0.01011890082499286928, 0.01079340861340093508, 0.01146791640180900088, 0.01214242419021706668, 0.01281693197862512901, 0.01349143976703319481 ),
 .UNSPECIFIED. ) ;
#16416=CARTESIAN_POINT ( 'NONE',  ( 2.646962709418357207, -0.2171425501261921576, 50.59379564821414732 ) ) ;
#16422=CARTESIAN_POINT ( 'NONE',  ( -36.44155368744861079, 56.74635804676026396, 22.50216374311547440 ) ) ;
#16425=DIRECTION ( 'NONE',  ( 1.558623840612994987E-16, 1.000000000000000000, 0.000000000000000000 ) ) ;
#16426=DIRECTION ( 'NONE',  ( 0.000000000000000000, 0.000000000000000000, 1.000000000000000000 ) ) ;
#16429=FACE_BOUND ( 'NONE', #1639, .T. ) ;
#16433=ORIENTED_EDGE ( 'NONE', *, *, #7547, .F. ) ;
#16435=CARTESIAN_POINT ( 'NONE',  ( 276.3098885457529832, -32.62665103886256190, -7.000000000000010658 ) ) ;
#16439=CARTESIAN_POINT ( 'NONE',  ( -72.03667955647439669, 58.95149196695728477, 22.49965440599313737 ) ) ;
#16443=VECTOR ( 'NONE', #6393, 1000.000000000000000 ) ;
#16445=DIRECTION ( 'NONE',  ( -0.000000000000000000, -0.000000000000000000, -1.000000000000000000 ) ) ;
#16447=ORIENTED_EDGE ( 'NONE', *, *, #890, .T. ) ;
#16448=EDGE_CURVE ( 'NONE', #3111, #10621, #2193, .T. ) ;
#16450=FACE_OUTER_BOUND ( 'NONE', #12565, .T. ) ;
#16453=AXIS2_PLACEMENT_3D ( 'NONE', #7506, #3287, #11994 ) ;
#16463=DIRECTION ( 'NONE',  ( 0.000000000000000000, 0.000000000000000000, 1.000000000000000000 ) ) ;
#16465=CARTESIAN_POINT ( 'NONE',  ( -47.49688818721907069, 51.11831089686643281, -26.54642412129686946 ) ) ;
#16474=CARTESIAN_POINT ( 'NONE',  ( -66.40868851600848188, 112.0764521540501875, 25.00000000000000355 ) ) ;
#16485=VERTEX_POINT ( 'NONE', #16122 ) ;
#16496=AXIS2_PLACEMENT_3D ( 'NONE', #12402, #9773, #1258 ) ;
#16504=DIRECTION ( 'NONE',  ( 1.119176436114069332E-16, -1.000000000000000000, -0.000000000000000000 ) ) ;
#16505=VERTEX_POINT ( 'NONE', #13615 ) ;
#16511=ORIENTED_EDGE ( 'NONE', *, *, #17048, .T. ) ;
#16517=CARTESIAN_POINT ( 'NONE',  ( -0.2223658127159511277, 8.412189173444385659, 47.97586337870632178 ) ) ;
#16522=CARTESIAN_POINT ( 'NONE',  ( -92.59262256747319952, 50.58224449241410525, 35.00000000000000000 ) ) ;
#16523=CARTESIAN_POINT ( 'NONE',  ( -32.61407059759434190, 55.22775151712274777, 23.63987630418073138 ) ) ;
#16524=ORIENTED_EDGE ( 'NONE', *, *, #5589, .T. ) ;
#16530=AXIS2_PLACEMENT_3D ( 'NONE', #7085, #1383, #9792 ) ;
#16532=ORIENTED_EDGE ( 'NONE', *, *, #15713, .T. ) ;
#16534=EDGE_LOOP ( 'NONE', ( #11008, #14348, #11734, #4946, #5008, #12308, #12110 ) ) ;
#16538=CARTESIAN_POINT ( 'NONE',  ( -72.85080879164550538, 59.45131026333987023, 22.67300586969097154 ) ) ;
#16539=CARTESIAN_POINT ( 'NONE',  ( -67.37428258903915435, 61.13748432492121765, -28.00000000000000000 ) ) ;
#16540=DIRECTION ( 'NONE',  ( 0.000000000000000000, 0.000000000000000000, 1.000000000000000000 ) ) ;
#16546=EDGE_CURVE ( 'NONE', #12660, #3213, #9408, .T. ) ;
#16550=CIRCLE ( 'NONE', #13573, 3.999999999999989786 ) ;
#16551=DIRECTION ( 'NONE',  ( 0.000000000000000000, -1.000000000000000000, 4.000800291689476254E-17 ) ) ;
#16559=UNCERTAINTY_MEASURE_WITH_UNIT (LENGTH_MEASURE( 1.000000000000000082E-05 ), #443, 'distance_accuracy_value', 'NONE');
#16560=FACE_OUTER_BOUND ( 'NONE', #4124, .T. ) ;
#16562=DIRECTION ( 'NONE',  ( 0.000000000000000000, 0.000000000000000000, 1.000000000000000000 ) ) ;
#16564=CARTESIAN_POINT ( 'NONE',  ( 79.02261728059691848, -151.5628872026273086, -57.00000000000000000 ) ) ;
#16570=DIRECTION ( 'NONE',  ( 1.000000000000000000, -0.000000000000000000, 5.204170427930409450E-16 ) ) ;
#16574=DIRECTION ( 'NONE',  ( -0.000000000000000000, -0.000000000000000000, -1.000000000000000000 ) ) ;
#16579=EDGE_LOOP ( 'NONE', ( #2620, #13649 ) ) ;
#16580=ADVANCED_FACE ( 'NONE', ( #1370 ), #6686, .T. ) ;
#16586=LINE ( 'NONE', #9477, #9694 ) ;
#16600=CARTESIAN_POINT ( 'NONE',  ( -74.72098969274614433, 107.7097065371563502, -23.55747138529295981 ) ) ;
#16601=CARTESIAN_POINT ( 'NONE',  ( -66.14689449588691161, 109.7265287073793871, 25.00000000000000000 ) ) ;
#16613=DIRECTION ( 'NONE',  ( 0.000000000000000000, 0.000000000000000000, 1.000000000000000000 ) ) ;
#16619=CARTESIAN_POINT ( 'NONE',  ( -21.95659417082859832, 49.25911447477409411, 27.80848509855457351 ) ) ;
#16620=ORIENTED_EDGE ( 'NONE', *, *, #13065, .T. ) ;
#16629=VERTEX_POINT ( 'NONE', #16676 ) ;
#16630=CARTESIAN_POINT ( 'NONE',  ( -64.09025127992791226, 117.8748711238780373, 35.00000000000000000 ) ) ;
#16634=CARTESIAN_POINT ( 'NONE',  ( -127.5926225674731995, 110.5691553257988460, -30.35917033480641081 ) ) ;
#16645=ORIENTED_EDGE ( 'NONE', *, *, #3208, .T. ) ;
#16653=CARTESIAN_POINT ( 'NONE',  ( -66.75430539726967538, 111.9591114379528278, 24.14213053467310388 ) ) ;
#16664=EDGE_CURVE ( 'NONE', #11287, #4482, #17648, .T. ) ;
#16668=EDGE_CURVE ( 'NONE', #16505, #565, #2678, .T. ) ;
#16669=CYLINDRICAL_SURFACE ( 'NONE', #8752, 20.99999999999999645 ) ;
#16672=CARTESIAN_POINT ( 'NONE',  ( 9.725871859128035979, 10.18744197292029519, -47.32031891155416758 ) ) ;
#16673=CARTESIAN_POINT ( 'NONE',  ( 49.38736944425944841, -141.5628872026273086, 57.00000000000000000 ) ) ;
#16676=CARTESIAN_POINT ( 'NONE',  ( -66.51364668169601657, 56.41604328733773599, -28.00000000000000355 ) ) ;
#16680=ADVANCED_FACE ( 'NONE', ( #16971 ), #4162, .F. ) ;
#16687=CARTESIAN_POINT ( 'NONE',  ( -66.28571926091831301, 56.33965956596666302, -25.37336305160129157 ) ) ;
#16696=DIRECTION ( 'NONE',  ( -0.000000000000000000, -0.000000000000000000, -1.000000000000000000 ) ) ;
#16698=VECTOR ( 'NONE', #10413, 1000.000000000000000 ) ;
#16707=EDGE_CURVE ( 'NONE', #13442, #6499, #14451, .T. ) ;
#16713=VERTEX_POINT ( 'NONE', #302 ) ;
#16715=ORIENTED_EDGE ( 'NONE', *, *, #244, .T. ) ;
#16720=CARTESIAN_POINT ( 'NONE',  ( -66.33181866704592267, 58.86497344968405798, -28.00000000000000355 ) ) ;
#16724=ORIENTED_EDGE ( 'NONE', *, *, #12500, .F. ) ;
#16733=ORIENTED_EDGE ( 'NONE', *, *, #2932, .T. ) ;
#16739=VECTOR ( 'NONE', #17817, 1000.000000000000000 ) ;
#16749=DIRECTION ( 'NONE',  ( -0.000000000000000000, -0.000000000000000000, 1.000000000000000000 ) ) ;
#16757=ORIENTED_EDGE ( 'NONE', *, *, #15194, .F. ) ;
#16761=ORIENTED_EDGE ( 'NONE', *, *, #4410, .F. ) ;
#16771=CARTESIAN_POINT ( 'NONE',  ( 10.78549404122980881, 7.287009583740910124, -48.30585852359873655 ) ) ;
#16774=CYLINDRICAL_SURFACE ( 'NONE', #2120, 12.58237727243326987 ) ;
#16785=CARTESIAN_POINT ( 'NONE',  ( -66.42472841157137964, 56.38588342787130614, -27.77414277107697060 ) ) ;
#16789=ORIENTED_EDGE ( 'NONE', *, *, #6879, .F. ) ;
#16792=DIRECTION ( 'NONE',  ( 1.000000000000000000, 0.000000000000000000, 0.000000000000000000 ) ) ;
#16796=ORIENTED_EDGE ( 'NONE', *, *, #8934, .F. ) ;
#16797=DIRECTION ( 'NONE',  ( -0.000000000000000000, -0.000000000000000000, -1.000000000000000000 ) ) ;
#16807=CARTESIAN_POINT ( 'NONE',  ( -31.22998185749533206, 43.19966384034746198, -31.68386395162817237 ) ) ;
#16811=ADVANCED_FACE ( 'NONE', ( #12971 ), #7342, .F. ) ;
#16814=AXIS2_PLACEMENT_3D ( 'NONE', #18074, #5434, #6551 ) ;
#16815=DIRECTION ( 'NONE',  ( 1.000000000000000000, 0.000000000000000000, 5.204170427930409450E-16 ) ) ;
#16817=EDGE_LOOP ( 'NONE', ( #17792, #5544, #12824, #559 ) ) ;
#16820=VECTOR ( 'NONE', #12645, 1000.000000000000000 ) ;
#16829=CARTESIAN_POINT ( 'NONE',  ( -66.40868851600845346, 56.38066346224191960, 25.00000000000000355 ) ) ;
#16834=FACE_OUTER_BOUND ( 'NONE', #8033, .T. ) ;
#16841=ORIENTED_EDGE ( 'NONE', *, *, #2983, .F. ) ;
#16842=LINE ( 'NONE', #18449, #3891 ) ;
#16844=ORIENTED_EDGE ( 'NONE', *, *, #6514, .T. ) ;
#16857=CARTESIAN_POINT ( 'NONE',  ( -86.44887054343442401, 84.22855780814606419, 37.50000000000000000 ) ) ;
#16867=ORIENTED_EDGE ( 'NONE', *, *, #15466, .F. ) ;
#16869=DIRECTION ( 'NONE',  ( 0.000000000000000000, 0.000000000000000000, 1.000000000000000000 ) ) ;
#16872=VECTOR ( 'NONE', #18114, 1000.000000000000000 ) ;
#16878=DIRECTION ( 'NONE',  ( -0.000000000000000000, -0.000000000000000000, -1.000000000000000000 ) ) ;
#16883=LINE ( 'NONE', #4079, #6334 ) ;
#16894=AXIS2_PLACEMENT_3D ( 'NONE', #3434, #17832, #17547 ) ;
#16900=DIRECTION ( 'NONE',  ( 1.000000000000000000, 0.000000000000000000, 0.000000000000000000 ) ) ;
#16902=CARTESIAN_POINT ( 'NONE',  ( -21.29915789792537240, 36.55190282534568524, 35.57109117979849344 ) ) ;
#16904=ORIENTED_EDGE ( 'NONE', *, *, #8590, .F. ) ;
#16906=PLANE ( 'NONE',  #1962 ) ;
#16910=CARTESIAN_POINT ( 'NONE',  ( -1.504738427136219414, 30.29321795796768058, 38.83614924640553312 ) ) ;
#16914=B_SPLINE_CURVE_WITH_KNOTS ( 'NONE', 3,
 ( #11002, #7079, #11295, #9978, #9695, #16687, #16980, #6882, #3978, #11199, #18303, #12705, #16785, #15489 ),
 .UNSPECIFIED., .F., .F.,
 ( 4, 2, 2, 2, 2, 2, 4 ),
 ( 0.0005070788824283136874, 0.001978938528116338819, 0.003450798173804364277, 0.004186727996648383077, 0.004922657819492402310, 0.005658587642336421544, 0.006394517465180440778 ),
 .UNSPECIFIED. ) ;
#16920=PLANE ( 'NONE',  #395 ) ;
#16929=CARTESIAN_POINT ( 'NONE',  ( -66.56703568903412815, 108.9611403144850783, -28.00000000000000355 ) ) ;
#16936=EDGE_CURVE ( 'NONE', #2809, #7618, #14979, .T. ) ;
#16942=EDGE_CURVE ( 'NONE', #10632, #11429, #10219, .T. ) ;
#16945=EDGE_CURVE ( 'NONE', #13490, #885, #6177, .T. ) ;
#16946=EDGE_CURVE ( 'NONE', #996, #9439, #6935, .T. ) ;
#16947=EDGE_CURVE ( 'NONE', #8038, #16154, #6847, .T. ) ;
#16959=LINE ( 'NONE', #11068, #13104 ) ;
#16969=ORIENTED_EDGE ( 'NONE', *, *, #18181, .F. ) ;
#16971=FACE_OUTER_BOUND ( 'NONE', #16534, .T. ) ;
#16973=EDGE_LOOP ( 'NONE', ( #3101, #11350, #15975, #10365 ) ) ;
#16980=CARTESIAN_POINT ( 'NONE',  ( -66.22404118522587169, 56.31946035176153487, -25.60950434884761506 ) ) ;
#16981=VERTEX_POINT ( 'NONE', #3947 ) ;
#16986=ORIENTED_EDGE ( 'NONE', *, *, #14769, .F. ) ;
#16987=B_SPLINE_CURVE_WITH_KNOTS ( 'NONE', 3,
 ( #12648, #18346, #2814, #9918, #11418, #8321, #5518, #11244, #16929, #5690, #2713, #15521, #7027, #1410 ),
 .UNSPECIFIED., .F., .F.,
 ( 4, 2, 2, 2, 2, 2, 4 ),
 ( 0.01773859478439106935, 0.01909689306834340405, 0.01977604221031956794, 0.02045519135229573529, 0.02113434049427189917, 0.02181348963624806653, 0.02317178792020043246 ),
 .UNSPECIFIED. ) ;
#16997=CARTESIAN_POINT ( 'NONE',  ( -28.63941924468362998, 41.66079135237048803, -32.61277883979558823 ) ) ;
#17008=ORIENTED_EDGE ( 'NONE', *, *, #12825, .F. ) ;
#17010=CARTESIAN_POINT ( 'NONE',  ( -75.86129610575210336, 61.64996188551982925, 25.00000000000000355 ) ) ;
#17011=CARTESIAN_POINT ( 'NONE',  ( -57.08002265617300708, 84.22855780814606419, -47.49999999999999289 ) ) ;
#17014=DIRECTION ( 'NONE',  ( 0.000000000000000000, 0.000000000000000000, 1.000000000000000000 ) ) ;
#17016=LINE ( 'NONE', #13013, #6104 ) ;
#17025=CARTESIAN_POINT ( 'NONE',  ( -70.85175816390371040, -141.5628872026273086, -57.00000000000000000 ) ) ;
#17038=VECTOR ( 'NONE', #13933, 1000.000000000000000 ) ;
#17039=EDGE_LOOP ( 'NONE', ( #5321, #14760, #591, #10677 ) ) ;
#17048=EDGE_CURVE ( 'NONE', #16981, #4466, #11063, .T. ) ;
#17053=AXIS2_PLACEMENT_3D ( 'NONE', #2787, #16797, #12325 ) ;
#17056=CARTESIAN_POINT ( 'NONE',  ( -100.4870060002411805, -151.5628872026273086, 57.00000000000000000 ) ) ;
#17065=CARTESIAN_POINT ( 'NONE',  ( -102.4618227840623774, -151.5628872026273086, -36.00000000000000000 ) ) ;
#17077=AXIS2_PLACEMENT_3D ( 'NONE', #11707, #16003, #3188 ) ;
#17081=AXIS2_PLACEMENT_3D ( 'NONE', #9257, #16357, #17667 ) ;
#17084=ORIENTED_EDGE ( 'NONE', *, *, #4597, .F. ) ;
#17086=CARTESIAN_POINT ( 'NONE',  ( -50.41499038512538533, 117.9449492212793444, -7.000000000000013323 ) ) ;
#17093=CARTESIAN_POINT ( 'NONE',  ( 11.11858012585388522, 6.298571833544852616, 48.62870262240658548 ) ) ;
#17107=AXIS2_PLACEMENT_3D ( 'NONE', #3209, #8748, #7608 ) ;
#17115=ORIENTED_EDGE ( 'NONE', *, *, #11817, .T. ) ;
#17118=CARTESIAN_POINT ( 'NONE',  ( -123.4618227840623632, -151.5628872026273086, 36.00000000000000711 ) ) ;
#17119=VERTEX_POINT ( 'NONE', #11949 ) ;
#17126=VECTOR ( 'NONE', #5102, 1000.000000000000000 ) ;
#17137=DIRECTION ( 'NONE',  ( -0.000000000000000000, 0.000000000000000000, -1.000000000000000000 ) ) ;
#17140=PLANE ( 'NONE',  #17614 ) ;
#17149=CARTESIAN_POINT ( 'NONE',  ( -102.4618227840623774, -151.5628872026273086, -57.00000000000000000 ) ) ;
#17152=EDGE_CURVE ( 'NONE', #3088, #13411, #17373, .T. ) ;
#17153=CIRCLE ( 'NONE', #1027, 26.04359719766049608 ) ;
#17163=DIRECTION ( 'NONE',  ( -1.000000000000000000, 0.000000000000000000, 0.000000000000000000 ) ) ;
#17172=EDGE_CURVE ( 'NONE', #13472, #15291, #8106, .T. ) ;
#17178=EDGE_CURVE ( 'NONE', #4, #18453, #3056, .T. ) ;
#17182=CYLINDRICAL_SURFACE ( 'NONE', #9229, 11.04359719766049430 ) ;
#17184=CARTESIAN_POINT ( 'NONE',  ( 276.3098885457529832, -32.62665103886256190, -7.000000000000010658 ) ) ;
#17194=FACE_OUTER_BOUND ( 'NONE', #13548, .T. ) ;
#17198=VERTEX_POINT ( 'NONE', #8013 ) ;
#17199=CARTESIAN_POINT ( 'NONE',  ( -123.4618227840623632, -151.5628872026273086, -35.99999999999997158 ) ) ;
#17203=CARTESIAN_POINT ( 'NONE',  ( -67.59262256747315689, 111.6514400295689313, 15.00000000000006040 ) ) ;
#17208=CARTESIAN_POINT ( 'NONE',  ( -194.4437806548868934, -151.5628872026273086, 18.23991632971911869 ) ) ;
#17224=EDGE_CURVE ( 'NONE', #2102, #8537, #6610, .T. ) ;
#17225=DIRECTION ( 'NONE',  ( 1.000000000000000000, 0.000000000000000000, 0.000000000000000000 ) ) ;
#17231=EDGE_LOOP ( 'NONE', ( #9317, #4454, #12485, #11241, #1040, #5770, #12805 ) ) ;
#17235=B_SPLINE_CURVE_WITH_KNOTS ( 'NONE', 3,
 ( #10172, #7192, #2979, #1749, #13175, #4647, #11766, #8685, #11590, #15622, #8521, #11415, #10011, #2902 ),
 .UNSPECIFIED., .F., .F.,
 ( 4, 2, 2, 2, 2, 2, 4 ),
 ( 0.0006178928065812205276, 0.001352643563036826091, 0.002087394319492431871, 0.002822145075948037651, 0.003556895832403643432, 0.005026397345314864533, 0.006495898858226086502 ),
 .UNSPECIFIED. ) ;
#17238=VERTEX_POINT ( 'NONE', #632 ) ;
#17244=CARTESIAN_POINT ( 'NONE',  ( 15.23320273812466041, 0.000000000000000000, 3.000000000000000000 ) ) ;
#17246=LINE ( 'NONE', #7156, #10441 ) ;
#17251=DIRECTION ( 'NONE',  ( 0.000000000000000000, 0.000000000000000000, 1.000000000000000000 ) ) ;
#17254=VERTEX_POINT ( 'NONE', #3438 ) ;
#17262=EDGE_CURVE ( 'NONE', #16485, #1951, #4538, .T. ) ;
#17265=DIRECTION ( 'NONE',  ( -0.9475106458593564041, -0.3197242186372270534, 0.000000000000000000 ) ) ;
#17275=EDGE_CURVE ( 'NONE', #9163, #11177, #18485, .T. ) ;
#17285=ADVANCED_FACE ( 'NONE', ( #2607 ), #14212, .F. ) ;
#17295=ORIENTED_EDGE ( 'NONE', *, *, #931, .T. ) ;
#17302=FACE_OUTER_BOUND ( 'NONE', #18380, .T. ) ;
#17304=VERTEX_POINT ( 'NONE', #18503 ) ;
#17308=VECTOR ( 'NONE', #4969, 1000.000000000000000 ) ;
#17317=AXIS2_PLACEMENT_3D ( 'NONE', #9081, #4583, #13372 ) ;
#17319=CARTESIAN_POINT ( 'NONE',  ( -67.59262256747315689, 56.80567558672318285, 15.00000000000006928 ) ) ;
#17323=ORIENTED_EDGE ( 'NONE', *, *, #11920, .T. ) ;
#17343=DIRECTION ( 'NONE',  ( -1.000000000000000000, -0.000000000000000000, -0.000000000000000000 ) ) ;
#17358=ORIENTED_EDGE ( 'NONE', *, *, #5610, .F. ) ;
#17362=CARTESIAN_POINT ( 'NONE',  ( -67.59262256747317110, 57.88796029049329661, 30.35917033480639660 ) ) ;
#17373=LINE ( 'NONE', #7652, #12917 ) ;
#17375=ORIENTED_EDGE ( 'NONE', *, *, #1762, .F. ) ;
#17377=AXIS2_PLACEMENT_3D ( 'NONE', #12013, #6386, #11917 ) ;
#17383=VECTOR ( 'NONE', #5861, 1000.000000000000000 ) ;
#17385=EDGE_CURVE ( 'NONE', #9318, #6499, #11843, .T. ) ;
#17401=CARTESIAN_POINT ( 'NONE',  ( -92.59262256747321373, 110.5691553257988460, 30.35917033480641081 ) ) ;
#17405=VERTEX_POINT ( 'NONE', #10255 ) ;
#17410=AXIS2_PLACEMENT_3D ( 'NONE', #11588, #10266, #3163 ) ;
#17419=DIRECTION ( 'NONE',  ( 0.000000000000000000, 1.000000000000000000, -0.000000000000000000 ) ) ;
#17420=EDGE_LOOP ( 'NONE', ( #16645, #8696, #4381, #6353, #7554 ) ) ;
#17425=LINE ( 'NONE', #14619, #12589 ) ;
#17427=ORIENTED_EDGE ( 'NONE', *, *, #7769, .T. ) ;
#17434=ORIENTED_EDGE ( 'NONE', *, *, #116, .T. ) ;
#17438=VECTOR ( 'NONE', #5643, 1000.000000000000000 ) ;
#17451=VECTOR ( 'NONE', #8180, 1000.000000000000000 ) ;
#17452=ORIENTED_EDGE ( 'NONE', *, *, #331, .F. ) ;
#17455=ADVANCED_FACE ( 'NONE', ( #170 ), #8773, .F. ) ;
#17464=ORIENTED_EDGE ( 'NONE', *, *, #15703, .T. ) ;
#17473=ORIENTED_EDGE ( 'NONE', *, *, #757, .F. ) ;
#17478=EDGE_CURVE ( 'NONE', #7906, #2272, #17532, .T. ) ;
#17490=ORIENTED_EDGE ( 'NONE', *, *, #10532, .F. ) ;
#17500=ORIENTED_EDGE ( 'NONE', *, *, #15466, .T. ) ;
#17507=FACE_BOUND ( 'NONE', #7119, .T. ) ;
#17512=CARTESIAN_POINT ( 'NONE',  ( -66.20428811384469725, 111.5958523346568967, 25.00000000000000711 ) ) ;
#17517=EDGE_CURVE ( 'NONE', #15284, #4575, #2756, .T. ) ;
#17527=CARTESIAN_POINT ( 'NONE',  ( -57.08002265617300708, 84.22855780814606419, -28.00000000000000355 ) ) ;
#17532=LINE ( 'NONE', #2966, #17383 ) ;
#17543=FACE_OUTER_BOUND ( 'NONE', #11387, .T. ) ;
#17547=DIRECTION ( 'NONE',  ( 1.000000000000000000, 0.000000000000000000, 0.000000000000000000 ) ) ;
#17553=SHAPE_REPRESENTATION ( 'C-Frame Forged Steel Casing', ( #16217 ), #2819 ) ;
#17563=DIRECTION ( 'NONE',  ( 1.000000000000000000, 0.000000000000000000, 0.000000000000000000 ) ) ;
#17564=CARTESIAN_POINT ( 'NONE',  ( 103.5381772159376084, -111.0842361345572158, -57.00000000000000000 ) ) ;
#17573=FACE_OUTER_BOUND ( 'NONE', #5407, .T. ) ;
#17578=CARTESIAN_POINT ( 'NONE',  ( 15.23320273812467462, -111.0842361345572158, 57.00000000000000000 ) ) ;
#17580=EDGE_CURVE ( 'NONE', #11429, #6748, #13975, .T. ) ;
#17588=VECTOR ( 'NONE', #1105, 1000.000000000000114 ) ;
#17600=ORIENTED_EDGE ( 'NONE', *, *, #12238, .F. ) ;
#17604=ADVANCED_FACE ( 'NONE', ( #3590, #3408, #4993 ), #12125, .F. ) ;
#17609=PLANE ( 'NONE',  #13889 ) ;
#17614=AXIS2_PLACEMENT_3D ( 'NONE', #2740, #4328, #1521 ) ;
#17622=DIRECTION ( 'NONE',  ( 1.000000000000000000, 0.000000000000000000, 0.000000000000000000 ) ) ;
#17632=VECTOR ( 'NONE', #8675, 1000.000000000000000 ) ;
#17643=DIRECTION ( 'NONE',  ( 4.124608743189000987E-16, -1.000000000000000000, 0.000000000000000000 ) ) ;
#17648=CIRCLE ( 'NONE', #11101, 180.8515291679561585 ) ;
#17660=AXIS2_PLACEMENT_3D ( 'NONE', #11995, #680, #7507 ) ;
#17663=DIRECTION ( 'NONE',  ( 0.000000000000000000, 0.000000000000000000, -1.000000000000000000 ) ) ;
#17664=CARTESIAN_POINT ( 'NONE',  ( -71.49209981491081578, 109.8200333694789776, 22.42650986270964353 ) ) ;
#17667=DIRECTION ( 'NONE',  ( -1.000000000000000000, 0.000000000000000000, -0.000000000000000000 ) ) ;
#17669=CARTESIAN_POINT ( 'NONE',  ( 105.4583593777967963, -32.62665103886256190, 7.000000000000010658 ) ) ;
#17674=DIRECTION ( 'NONE',  ( 0.000000000000000000, 0.000000000000000000, 1.000000000000000000 ) ) ;
#17686=EDGE_LOOP ( 'NONE', ( #5592, #5079 ) ) ;
#17689=AXIS2_PLACEMENT_3D ( 'NONE', #8447, #8265, #9765 ) ;
#17702=CARTESIAN_POINT ( 'NONE',  ( -27.71117476891160081, 84.22855780814606419, -28.00000000000000355 ) ) ;
#17716=DIRECTION ( 'NONE',  ( 1.000000000000000000, 2.062304371594500494E-16, -0.000000000000000000 ) ) ;
#17722=CIRCLE ( 'NONE', #412, 18.23991632971911514 ) ;
#17723=EDGE_CURVE ( 'NONE', #7906, #1253, #8288, .T. ) ;
#17725=CARTESIAN_POINT ( 'NONE',  ( -67.42362413453201953, 107.1062079628228503, 25.00000000000000000 ) ) ;
#17735=AXIS2_PLACEMENT_3D ( 'NONE', #17184, #15775, #3993 ) ;
#17749=CARTESIAN_POINT ( 'NONE',  ( -9.409811683556181805, 39.33212575317277526, 34.01304937313500432 ) ) ;
#17760=CARTESIAN_POINT ( 'NONE',  ( -123.4618227840623632, -111.0842361345572158, 57.00000000000000000 ) ) ;
#17762=VERTEX_POINT ( 'NONE', #11194 ) ;
#17764=DIRECTION ( 'NONE',  ( -1.000000000000000000, 0.000000000000000000, 0.000000000000000000 ) ) ;
#17771=LINE ( 'NONE', #9256, #4342 ) ;
#17772=CARTESIAN_POINT ( 'NONE',  ( 0.000000000000000000, 0.000000000000000000, -57.00000000000000000 ) ) ;
#17774=CARTESIAN_POINT ( 'NONE',  ( -75.66356596311996441, 61.48658486655093469, -24.60062213568815537 ) ) ;
#17784=CARTESIAN_POINT ( 'NONE',  ( -86.44887054343442401, 84.22855780814606419, -28.00000000000000355 ) ) ;
#17787=ORIENTED_EDGE ( 'NONE', *, *, #5830, .T. ) ;
#17792=ORIENTED_EDGE ( 'NONE', *, *, #8148, .F. ) ;
#17799=ORIENTED_EDGE ( 'NONE', *, *, #10650, .F. ) ;
#17807=LINE ( 'NONE', #7805, #2728 ) ;
#17817=DIRECTION ( 'NONE',  ( 1.000000000000000000, 1.119176436114069332E-16, 0.000000000000000000 ) ) ;
#17819=ORIENTED_EDGE ( 'NONE', *, *, #11548, .F. ) ;
#17823=DIRECTION ( 'NONE',  ( 1.000000000000000000, 0.000000000000000000, 0.000000000000000000 ) ) ;
#17832=DIRECTION ( 'NONE',  ( -0.000000000000000000, -0.000000000000000000, 1.000000000000000000 ) ) ;
#17845=ORIENTED_EDGE ( 'NONE', *, *, #7223, .F. ) ;
#17851=DIRECTION ( 'NONE',  ( -0.000000000000000000, -0.000000000000000000, -1.000000000000000000 ) ) ;
#17852=CARTESIAN_POINT ( 'NONE',  ( -70.06856178257687873, 57.88796029049330372, 22.35917033480642502 ) ) ;
#17854=DIRECTION ( 'NONE',  ( -1.000000000000000000, 0.000000000000000000, 0.000000000000000000 ) ) ;
#17857=ORIENTED_EDGE ( 'NONE', *, *, #1063, .T. ) ;
#17858=CARTESIAN_POINT ( 'NONE',  ( -72.80844527697490776, 59.42543905650232716, -22.66411427748654361 ) ) ;
#17859=CARTESIAN_POINT ( 'NONE',  ( -86.44887054343442401, 84.22855780814606419, 25.00000000000000355 ) ) ;
#17865=ORIENTED_EDGE ( 'NONE', *, *, #2544, .F. ) ;
#17871=VERTEX_POINT ( 'NONE', #9547 ) ;
#17892=DIRECTION ( 'NONE',  ( 0.000000000000000000, 1.000000000000000000, 0.000000000000000000 ) ) ;
#17893=LINE ( 'NONE', #11185, #17451 ) ;
#17899=CARTESIAN_POINT ( 'NONE',  ( 276.3098885457529832, -32.62665103886256190, 7.000000000000010658 ) ) ;
#17910=EDGE_LOOP ( 'NONE', ( #263, #5205, #9068, #13027, #3315 ) ) ;
#17914=DIRECTION ( 'NONE',  ( 0.000000000000000000, 1.000000000000000000, 0.000000000000000000 ) ) ;
#17916=CARTESIAN_POINT ( 'NONE',  ( 1.461703886464493563, 3.647763842320571825, 49.46183131592236037 ) ) ;
#17917=DIRECTION ( 'NONE',  ( -1.000000000000000000, 2.826528109797569363E-15, 0.000000000000000000 ) ) ;
#17921=DIRECTION ( 'NONE',  ( -0.5150380749100562650, 0.000000000000000000, 0.8571673007021111124 ) ) ;
#17933=EDGE_LOOP ( 'NONE', ( #17323, #9778 ) ) ;
#17941=DIRECTION ( 'NONE',  ( -0.000000000000000000, 0.000000000000000000, 1.000000000000000000 ) ) ;
#17951=PLANE ( 'NONE',  #3975 ) ;
#17952=FACE_OUTER_BOUND ( 'NONE', #6213, .T. ) ;
#17961=ORIENTED_EDGE ( 'NONE', *, *, #10104, .T. ) ;
#17977=ORIENTED_EDGE ( 'NONE', *, *, #12514, .T. ) ;
#17990=DIRECTION ( 'NONE',  ( -1.000000000000000000, -0.000000000000000000, -0.000000000000000000 ) ) ;
#17992=CARTESIAN_POINT ( 'NONE',  ( 124.5381772159375942, -151.5628872026272802, -35.99999999999997158 ) ) ;
#18000=DIRECTION ( 'NONE',  ( -0.000000000000000000, 0.000000000000000000, 1.000000000000000000 ) ) ;
#18001=LINE ( 'NONE', #6134, #3057 ) ;
#18003=CARTESIAN_POINT ( 'NONE',  ( -76.15046549741104798, 106.5634658120143570, -26.28507553062743085 ) ) ;
#18010=ORIENTED_EDGE ( 'NONE', *, *, #7011, .T. ) ;
#18011=AXIS2_PLACEMENT_3D ( 'NONE', #2300, #12430, #11015 ) ;
#18018=DIRECTION ( 'NONE',  ( 0.000000000000000000, 0.000000000000000000, 1.000000000000000000 ) ) ;
#18022=DIRECTION ( 'NONE',  ( -1.000000000000000000, 0.000000000000000000, 0.000000000000000000 ) ) ;
#18028=CARTESIAN_POINT ( 'NONE',  ( -1.859018761987631274, 12.02839362309843274, -46.70372576070108295 ) ) ;
#18034=DIRECTION ( 'NONE',  ( 0.000000000000000000, 0.000000000000000000, 1.000000000000000000 ) ) ;
#18045=CARTESIAN_POINT ( 'NONE',  ( -66.20417287045881949, 57.28139718322722018, -28.00000000000000711 ) ) ;
#18050=CIRCLE ( 'NONE', #1916, 34.36884788726141693 ) ;
#18056=EDGE_LOOP ( 'NONE', ( #16841, #6440, #15639, #3916 ) ) ;
#18059=LINE ( 'NONE', #7860, #7335 ) ;
#18060=CARTESIAN_POINT ( 'NONE',  ( -70.06856178257687873, 57.88796029049330372, 22.35917033480642502 ) ) ;
#18065=VECTOR ( 'NONE', #17343, 1000.000000000000000 ) ;
#18066=VECTOR ( 'NONE', #12469, 1000.000000000000000 ) ;
#18070=CYLINDRICAL_SURFACE ( 'NONE', #5216, 18.23991632971910803 ) ;
#18074=CARTESIAN_POINT ( 'NONE',  ( -57.08002265617300708, 84.22855780814606419, 37.50000000000000000 ) ) ;
#18075=EDGE_CURVE ( 'NONE', #13442, #17198, #12558, .T. ) ;
#18076=CARTESIAN_POINT ( 'NONE',  ( 95.45835937779683888, -32.62665103886254059, 7.000000000000010658 ) ) ;
#18078=ORIENTED_EDGE ( 'NONE', *, *, #15322, .F. ) ;
#18083=VERTEX_POINT ( 'NONE', #5431 ) ;
#18103=CARTESIAN_POINT ( 'NONE',  ( 11.11671913661698774, 6.304244514274031097, -48.62687381527162955 ) ) ;
#18105=DIRECTION ( 'NONE',  ( 1.000000000000000000, 0.000000000000000000, 0.000000000000000000 ) ) ;
#18114=DIRECTION ( 'NONE',  ( 0.000000000000000000, 0.000000000000000000, -1.000000000000000000 ) ) ;
#18121=ADVANCED_FACE ( 'NONE', ( #3005 ), #375, .F. ) ;
#18132=CARTESIAN_POINT ( 'NONE',  ( 15.23320273812466041, -19.34983604512934363, 54.79921157549236455 ) ) ;
#18138=DIRECTION ( 'NONE',  ( -0.3197242186372270534, 0.9475106458593564041, 0.000000000000000000 ) ) ;
#18139=ORIENTED_EDGE ( 'NONE', *, *, #3925, .F. ) ;
#18143=DIRECTION ( 'NONE',  ( -1.000000000000000000, 0.000000000000000000, 0.000000000000000000 ) ) ;
#18149=LINE ( 'NONE', #6824, #14056 ) ;
#18150=CARTESIAN_POINT ( 'NONE',  ( -50.06979403241810900, 50.58224449241409104, 26.91246033477412425 ) ) ;
#18154=DIRECTION ( 'NONE',  ( -0.000000000000000000, 1.000000000000000000, 0.000000000000000000 ) ) ;
#18170=CARTESIAN_POINT ( 'NONE',  ( -67.37337372105014310, 111.7354893787529022, 22.91102204468130310 ) ) ;
#18181=EDGE_CURVE ( 'NONE', #1895, #4188, #7218, .T. ) ;
#18186=LINE ( 'NONE', #14170, #3344 ) ;
#18211=CARTESIAN_POINT ( 'NONE',  ( -70.71978124295696944, -111.0842361345572158, 5.204170427930421283E-15 ) ) ;
#18214=VERTEX_POINT ( 'NONE', #6065 ) ;
#18217=CARTESIAN_POINT ( 'NONE',  ( -34.72861478725227613, 45.17254440751388245, 30.47173447583816852 ) ) ;
#18226=CARTESIAN_POINT ( 'NONE',  ( -0.3127821567423632598, 28.68880187506458412, 39.62697943036548764 ) ) ;
#18227=ORIENTED_EDGE ( 'NONE', *, *, #9291, .T. ) ;
#18237=CARTESIAN_POINT ( 'NONE',  ( -75.21640136043859570, 61.12840431439423838, 24.01061398482676879 ) ) ;
#18238=CARTESIAN_POINT ( 'NONE',  ( -66.51364668169601657, 56.41604328733773599, -28.00000000000000355 ) ) ;
#18241=LINE ( 'NONE', #16634, #4915 ) ;
#18251=VERTEX_POINT ( 'NONE', #17564 ) ;
#18255=ORIENTED_EDGE ( 'NONE', *, *, #16546, .T. ) ;
#18258=DIRECTION ( 'NONE',  ( 1.000000000000000000, 0.000000000000000000, 0.000000000000000000 ) ) ;
#18261=CYLINDRICAL_SURFACE ( 'NONE', #16814, 26.04359719766049253 ) ;
#18264=ORIENTED_EDGE ( 'NONE', *, *, #8942, .F. ) ;
#18267=DIRECTION ( 'NONE',  ( 1.000000000000000000, 0.000000000000000000, 0.000000000000000000 ) ) ;
#18285=AXIS2_PLACEMENT_3D ( 'NONE', #13681, #5440, #13775 ) ;
#18287=CARTESIAN_POINT ( 'NONE',  ( 15.23320273812466041, -19.34983604512935429, 57.00000000000000000 ) ) ;
#18303=CARTESIAN_POINT ( 'NONE',  ( -66.21794066256015299, 56.31741075272766039, -27.07314213088852739 ) ) ;
#18307=ORIENTED_EDGE ( 'NONE', *, *, #3858, .F. ) ;
#18310=ORIENTED_EDGE ( 'NONE', *, *, #8452, .F. ) ;
#18312=CARTESIAN_POINT ( 'NONE',  ( 15.23320273812466041, -19.34983604512934363, -3.000000000000000000 ) ) ;
#18314=CARTESIAN_POINT ( 'NONE',  ( -7.963671022379969600, 22.16714537965745890, 42.62291292524223252 ) ) ;
#18318=EDGE_CURVE ( 'NONE', #10530, #12457, #10251, .T. ) ;
#18325=DIRECTION ( 'NONE',  ( -1.119176436114069332E-16, 1.000000000000000000, 0.000000000000000000 ) ) ;
#18342=CARTESIAN_POINT ( 'NONE',  ( -50.41499038512538533, 117.9449492212793302, 0.000000000000000000 ) ) ;
#18343=CARTESIAN_POINT ( 'NONE',  ( -64.09025127992791226, 117.8748711238780373, 35.00000000000000000 ) ) ;
#18345=EDGE_LOOP ( 'NONE', ( #482, #4772, #2952, #3326 ) ) ;
#18346=CARTESIAN_POINT ( 'NONE',  ( -66.34489626515157568, 111.6204860916741239, -28.00000000000000000 ) ) ;
#18351=ORIENTED_EDGE ( 'NONE', *, *, #9835, .T. ) ;
#18362=AXIS2_PLACEMENT_3D ( 'NONE', #15023, #8005, #9601 ) ;
#18374=DIRECTION ( 'NONE',  ( 0.000000000000000000, -1.000000000000000000, -0.000000000000000000 ) ) ;
#18376=AXIS2_PLACEMENT_3D ( 'NONE', #6325, #2034, #7736 ) ;
#18378=DIRECTION ( 'NONE',  ( 0.000000000000000000, 0.000000000000000000, 1.000000000000000000 ) ) ;
#18380=EDGE_LOOP ( 'NONE', ( #6813, #16761, #12759, #9545 ) ) ;
#18382=EDGE_CURVE ( 'NONE', #17405, #7351, #1896, .T. ) ;
#18383=EDGE_LOOP ( 'NONE', ( #13580, #11143, #12512, #4527 ) ) ;
#18407=ADVANCED_FACE ( 'NONE', ( #15433 ), #1123, .F. ) ;
#18420=CARTESIAN_POINT ( 'NONE',  ( 1.801461313472378700, 2.685927156466989096, -49.76172839322247654 ) ) ;
#18425=DIRECTION ( 'NONE',  ( -0.000000000000000000, -0.000000000000000000, -1.000000000000000000 ) ) ;
#18430=EDGE_CURVE ( 'NONE', #9555, #12621, #8317, .T. ) ;
#18442=CARTESIAN_POINT ( 'NONE',  ( -36.44155368744861079, 56.74635804676026396, 22.50216374311547440 ) ) ;
#18444=VERTEX_POINT ( 'NONE', #11239 ) ;
#18449=CARTESIAN_POINT ( 'NONE',  ( -127.5926225674731995, 110.5691553257988460, -22.35917033480641791 ) ) ;
#18452=B_SPLINE_CURVE_WITH_KNOTS ( 'NONE', 3,
 ( #14780, #1975, #7675, #13380, #556, #4857, #10578, #14865, #2056, #7758, #14951, #13475, #656, #17774, #4958, #16359, #3546, #9262, #2146, #7855, #758, #6449, #12169, #17858, #5040, #12459, #15241, #6828 ),
 .UNSPECIFIED., .F., .F.,
 ( 4, 2, 2, 2, 2, 2, 2, 2, 2, 2, 2, 2, 2, 4 ),
 ( 0.000000000000000000, 0.0006831928620949466457, 0.001366385724189893291, 0.001707982155237364229, 0.002049578586284835167, 0.002732771448379764899, 0.003415964310474694197, 0.004099157172569624363, 0.004782350034664553662, 0.005465542896759482960, 0.006831928620949360639, 0.007515121483044319428, 0.008198314345139278217, 0.01093108579351914633 ),
 .UNSPECIFIED. ) ;
#18453=VERTEX_POINT ( 'NONE', #5686 ) ;
#18454=EDGE_CURVE ( 'NONE', #13683, #3387, #8230, .T. ) ;
#18465=FACE_OUTER_BOUND ( 'NONE', #4601, .T. ) ;
#18471=ORIENTED_EDGE ( 'NONE', *, *, #17172, .T. ) ;
#18472=CARTESIAN_POINT ( 'NONE',  ( -67.59262256747319952, 106.9211863004615140, -28.00000000000000355 ) ) ;
#18481=LINE ( 'NONE', #8285, #2794 ) ;
#18482=VERTEX_POINT ( 'NONE', #4552 ) ;
#18485=B_SPLINE_CURVE_WITH_KNOTS ( 'NONE', 3,
 ( #16422, #16523, #15028, #3721, #2306, #16619, #3812, #9514, #6323, #12051, #17749, #1114, #3901, #9607, #4287, #16910, #18226, #8304, #6901, #9713, #1471, #15422, #7178, #2888, #17093, #14114, #14018, #1302, #1391, #18132 ),
 .UNSPECIFIED., .F., .F.,
 ( 4, 2, 2, 2, 2, 2, 2, 2, 2, 2, 2, 2, 2, 2, 4 ),
 ( 0.01212337847808446674, 0.02493713703494332412, 0.02814057667415803543, 0.03134401631337273980, 0.03775089559180216936, 0.05056465414866103542, 0.05376809378787574673, 0.05697153342709045803, 0.06337841270551984596, 0.07619217126237863569, 0.08259905054080803055, 0.08580249018002272798, 0.08900592981923741154, 0.1018196883760962013, 0.1146334469329549632 ),
 .UNSPECIFIED. ) ;
#18494=ORIENTED_EDGE ( 'NONE', *, *, #12204, .F. ) ;
#18503=CARTESIAN_POINT ( 'NONE',  ( -83.12361985383351737, 84.22855780814606419, 35.00000000000000000 ) ) ;
#18506=CARTESIAN_POINT ( 'NONE',  ( 9.543663295069050534, 56.41207303426870112, -3.000000000000000000 ) ) ;
#18510=ORIENTED_EDGE ( 'NONE', *, *, #11249, .F. ) ;
#18532=COLOUR_RGB('Dark Blue',0.08,0.2,0.34);
#18533=FILL_AREA_STYLE_COLOUR('',#18532);
#18534=FILL_AREA_STYLE('',(#18533));
#18535=SURFACE_STYLE_FILL_AREA(#18534);
#18536=SURFACE_SIDE_STYLE('',(#18535));
#18537=SURFACE_STYLE_USAGE(.BOTH.,#18536);
#18538=PRESENTATION_STYLE_ASSIGNMENT((#18537));
ENDSEC;
END-ISO-10303-21;
